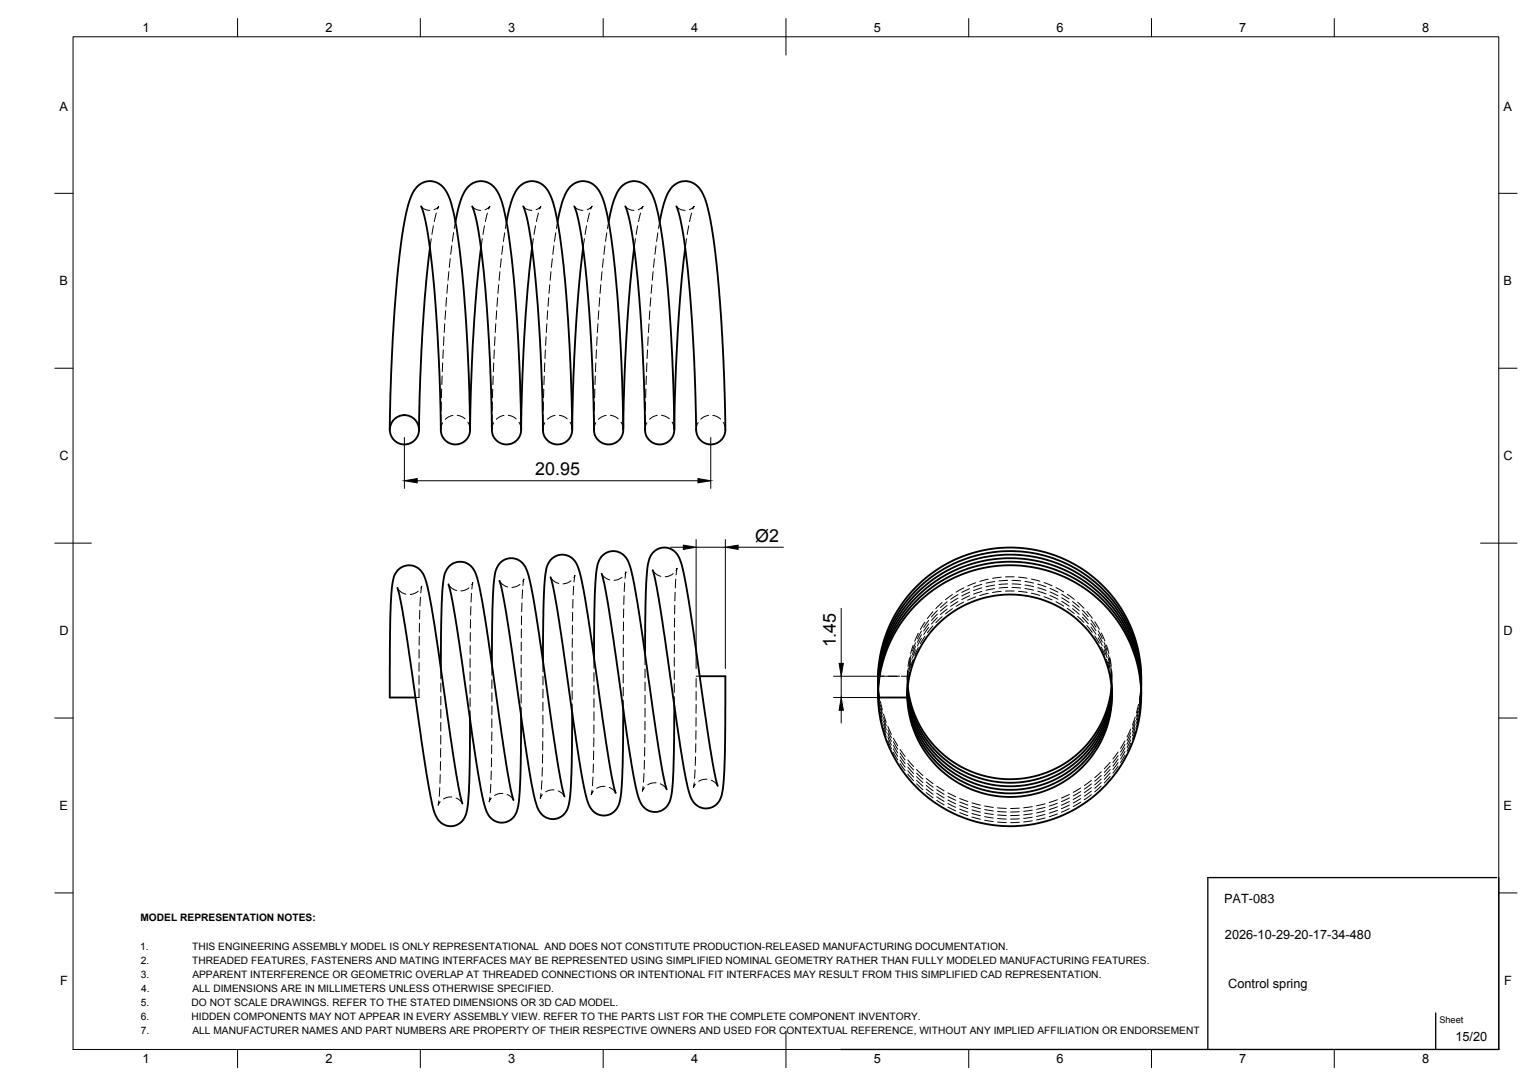
ISO-10303-21;
HEADER;
/* Generated by software containing ST-Developer
 * from STEP Tools, Inc. (www.steptools.com) 
 */

FILE_DESCRIPTION(
/* description */ ('PAT-083'),
/* implementation_level */ '2;1');

FILE_NAME(
/* name */ 'Control spring.step',
/* time_stamp */ '2026-10-29T20:18:00-07:00',
/* author */ (''),
/* organization */ (''),
/* preprocessor_version */ 'ST-DEVELOPER v20.2',
/* originating_system */ 'Autodesk Translation Framework v15.17.0.0',
/* authorisation */ '');

FILE_SCHEMA (('AUTOMOTIVE_DESIGN { 1 0 10303 214 3 1 1 }'));
ENDSEC;

DATA;
#10=MECHANICAL_DESIGN_GEOMETRIC_PRESENTATION_REPRESENTATION('',(#241),#8428);
#166=B_SPLINE_SURFACE_WITH_KNOTS('',3,3,((#7043,#7044,#7045,#7046,#7047,
#7048,#7049,#7050,#7051,#7052,#7053,#7054,#7055,#7056,#7057,#7058,#7059,
#7060,#7061,#7062,#7063,#7064,#7065,#7066,#7067,#7068,#7069,#7070,#7071,
#7072,#7073,#7074,#7075,#7076,#7077,#7078,#7079,#7080,#7081,#7082,#7083,
#7084,#7085,#7086,#7087,#7088,#7089,#7090,#7091,#7092,#7093,#7094,#7095,
#7096,#7097,#7098,#7099,#7100,#7101,#7102,#7103,#7104,#7105,#7106,#7107,
#7108,#7109,#7110,#7111,#7112,#7113),(#7114,#7115,#7116,#7117,#7118,#7119,
#7120,#7121,#7122,#7123,#7124,#7125,#7126,#7127,#7128,#7129,#7130,#7131,
#7132,#7133,#7134,#7135,#7136,#7137,#7138,#7139,#7140,#7141,#7142,#7143,
#7144,#7145,#7146,#7147,#7148,#7149,#7150,#7151,#7152,#7153,#7154,#7155,
#7156,#7157,#7158,#7159,#7160,#7161,#7162,#7163,#7164,#7165,#7166,#7167,
#7168,#7169,#7170,#7171,#7172,#7173,#7174,#7175,#7176,#7177,#7178,#7179,
#7180,#7181,#7182,#7183,#7184),(#7185,#7186,#7187,#7188,#7189,#7190,#7191,
#7192,#7193,#7194,#7195,#7196,#7197,#7198,#7199,#7200,#7201,#7202,#7203,
#7204,#7205,#7206,#7207,#7208,#7209,#7210,#7211,#7212,#7213,#7214,#7215,
#7216,#7217,#7218,#7219,#7220,#7221,#7222,#7223,#7224,#7225,#7226,#7227,
#7228,#7229,#7230,#7231,#7232,#7233,#7234,#7235,#7236,#7237,#7238,#7239,
#7240,#7241,#7242,#7243,#7244,#7245,#7246,#7247,#7248,#7249,#7250,#7251,
#7252,#7253,#7254,#7255),(#7256,#7257,#7258,#7259,#7260,#7261,#7262,#7263,
#7264,#7265,#7266,#7267,#7268,#7269,#7270,#7271,#7272,#7273,#7274,#7275,
#7276,#7277,#7278,#7279,#7280,#7281,#7282,#7283,#7284,#7285,#7286,#7287,
#7288,#7289,#7290,#7291,#7292,#7293,#7294,#7295,#7296,#7297,#7298,#7299,
#7300,#7301,#7302,#7303,#7304,#7305,#7306,#7307,#7308,#7309,#7310,#7311,
#7312,#7313,#7314,#7315,#7316,#7317,#7318,#7319,#7320,#7321,#7322,#7323,
#7324,#7325,#7326),(#7327,#7328,#7329,#7330,#7331,#7332,#7333,#7334,#7335,
#7336,#7337,#7338,#7339,#7340,#7341,#7342,#7343,#7344,#7345,#7346,#7347,
#7348,#7349,#7350,#7351,#7352,#7353,#7354,#7355,#7356,#7357,#7358,#7359,
#7360,#7361,#7362,#7363,#7364,#7365,#7366,#7367,#7368,#7369,#7370,#7371,
#7372,#7373,#7374,#7375,#7376,#7377,#7378,#7379,#7380,#7381,#7382,#7383,
#7384,#7385,#7386,#7387,#7388,#7389,#7390,#7391,#7392,#7393,#7394,#7395,
#7396,#7397),(#7398,#7399,#7400,#7401,#7402,#7403,#7404,#7405,#7406,#7407,
#7408,#7409,#7410,#7411,#7412,#7413,#7414,#7415,#7416,#7417,#7418,#7419,
#7420,#7421,#7422,#7423,#7424,#7425,#7426,#7427,#7428,#7429,#7430,#7431,
#7432,#7433,#7434,#7435,#7436,#7437,#7438,#7439,#7440,#7441,#7442,#7443,
#7444,#7445,#7446,#7447,#7448,#7449,#7450,#7451,#7452,#7453,#7454,#7455,
#7456,#7457,#7458,#7459,#7460,#7461,#7462,#7463,#7464,#7465,#7466,#7467,
#7468),(#7469,#7470,#7471,#7472,#7473,#7474,#7475,#7476,#7477,#7478,#7479,
#7480,#7481,#7482,#7483,#7484,#7485,#7486,#7487,#7488,#7489,#7490,#7491,
#7492,#7493,#7494,#7495,#7496,#7497,#7498,#7499,#7500,#7501,#7502,#7503,
#7504,#7505,#7506,#7507,#7508,#7509,#7510,#7511,#7512,#7513,#7514,#7515,
#7516,#7517,#7518,#7519,#7520,#7521,#7522,#7523,#7524,#7525,#7526,#7527,
#7528,#7529,#7530,#7531,#7532,#7533,#7534,#7535,#7536,#7537,#7538,#7539),
(#7540,#7541,#7542,#7543,#7544,#7545,#7546,#7547,#7548,#7549,#7550,#7551,
#7552,#7553,#7554,#7555,#7556,#7557,#7558,#7559,#7560,#7561,#7562,#7563,
#7564,#7565,#7566,#7567,#7568,#7569,#7570,#7571,#7572,#7573,#7574,#7575,
#7576,#7577,#7578,#7579,#7580,#7581,#7582,#7583,#7584,#7585,#7586,#7587,
#7588,#7589,#7590,#7591,#7592,#7593,#7594,#7595,#7596,#7597,#7598,#7599,
#7600,#7601,#7602,#7603,#7604,#7605,#7606,#7607,#7608,#7609,#7610),(#7611,
#7612,#7613,#7614,#7615,#7616,#7617,#7618,#7619,#7620,#7621,#7622,#7623,
#7624,#7625,#7626,#7627,#7628,#7629,#7630,#7631,#7632,#7633,#7634,#7635,
#7636,#7637,#7638,#7639,#7640,#7641,#7642,#7643,#7644,#7645,#7646,#7647,
#7648,#7649,#7650,#7651,#7652,#7653,#7654,#7655,#7656,#7657,#7658,#7659,
#7660,#7661,#7662,#7663,#7664,#7665,#7666,#7667,#7668,#7669,#7670,#7671,
#7672,#7673,#7674,#7675,#7676,#7677,#7678,#7679,#7680,#7681),(#7682,#7683,
#7684,#7685,#7686,#7687,#7688,#7689,#7690,#7691,#7692,#7693,#7694,#7695,
#7696,#7697,#7698,#7699,#7700,#7701,#7702,#7703,#7704,#7705,#7706,#7707,
#7708,#7709,#7710,#7711,#7712,#7713,#7714,#7715,#7716,#7717,#7718,#7719,
#7720,#7721,#7722,#7723,#7724,#7725,#7726,#7727,#7728,#7729,#7730,#7731,
#7732,#7733,#7734,#7735,#7736,#7737,#7738,#7739,#7740,#7741,#7742,#7743,
#7744,#7745,#7746,#7747,#7748,#7749,#7750,#7751,#7752)),.UNSPECIFIED.,.T.,
 .F.,.F.,(4,1,1,1,1,1,1,4),(4,1,1,1,1,1,1,1,1,1,1,1,1,1,1,1,1,1,1,1,1,1,
1,1,1,1,1,1,1,1,1,1,1,1,1,1,1,1,1,1,1,1,1,1,1,1,1,1,1,1,1,1,1,1,1,1,1,1,
1,1,1,1,1,1,1,1,1,1,4),(-3.14159265358979,-2.24399475256414,-1.34639685153848,
-0.448798950512828,0.448798950512828,1.34639685153848,2.24399475256414,
3.14159265358979),(0.,0.0178571428571429,0.0357142857142857,0.0535714285714286,
0.0714285714285714,0.0892857142857143,0.107142857142857,0.125,0.142857142857143,
0.150793650793651,0.158730158730159,0.174603174603175,0.19047619047619,
0.202380952380952,0.214285714285714,0.226190476190476,0.238095238095238,
0.25,0.261904761904762,0.267857142857143,0.273809523809524,0.285714285714286,
0.297619047619048,0.30952380952381,0.321428571428571,0.333333333333333,
0.349206349206349,0.365079365079365,0.380952380952381,0.396825396825397,
0.412698412698413,0.428571428571429,0.446428571428571,0.464285714285714,
0.476190476190476,0.488095238095238,0.5,0.517857142857143,0.535714285714286,
0.553571428571429,0.571428571428571,0.589285714285714,0.607142857142857,
0.625,0.642857142857143,0.660714285714286,0.678571428571428,0.696428571428571,
0.714285714285714,0.726190476190476,0.738095238095238,0.75,0.761904761904762,
0.773809523809524,0.785714285714286,0.797619047619047,0.809523809523809,
0.821428571428571,0.833333333333333,0.845238095238095,0.857142857142857,
0.875,0.892857142857143,0.910714285714286,0.928571428571429,0.946428571428571,
0.964285714285714,0.982142857142857,1.),.UNSPECIFIED.);
#177=B_SPLINE_CURVE_WITH_KNOTS('',3,(#7756,#7757,#7758,#7759,#7760,#7761,
#7762,#7763,#7764,#7765,#7766,#7767,#7768,#7769,#7770,#7771,#7772,#7773,
#7774,#7775,#7776,#7777,#7778,#7779,#7780,#7781,#7782,#7783,#7784,#7785,
#7786,#7787,#7788,#7789,#7790,#7791,#7792,#7793,#7794,#7795,#7796,#7797,
#7798,#7799,#7800,#7801,#7802,#7803,#7804,#7805,#7806,#7807,#7808,#7809,
#7810,#7811,#7812,#7813,#7814,#7815,#7816,#7817,#7818,#7819,#7820,#7821,
#7822,#7823,#7824,#7825,#7826),.UNSPECIFIED.,.F.,.F.,(4,1,1,1,1,1,1,1,1,
1,1,1,1,1,1,1,1,1,1,1,1,1,1,1,1,1,1,1,1,1,1,1,1,1,1,1,1,1,1,1,1,1,1,1,1,
1,1,1,1,1,1,1,1,1,1,1,1,1,1,1,1,1,1,1,1,1,1,1,4),(0.,0.0178571428571429,
0.0357142857142857,0.0535714285714286,0.0714285714285714,0.0892857142857143,
0.107142857142857,0.125,0.142857142857143,0.150793650793651,0.158730158730159,
0.174603174603175,0.19047619047619,0.202380952380952,0.214285714285714,
0.226190476190476,0.238095238095238,0.25,0.261904761904762,0.267857142857143,
0.273809523809524,0.285714285714286,0.297619047619048,0.30952380952381,
0.321428571428571,0.333333333333333,0.349206349206349,0.365079365079365,
0.380952380952381,0.396825396825397,0.412698412698413,0.428571428571429,
0.446428571428571,0.464285714285714,0.476190476190476,0.488095238095238,
0.5,0.517857142857143,0.535714285714286,0.553571428571429,0.571428571428571,
0.589285714285714,0.607142857142857,0.625,0.642857142857143,0.660714285714286,
0.678571428571428,0.696428571428571,0.714285714285714,0.726190476190476,
0.738095238095238,0.75,0.761904761904762,0.773809523809524,0.785714285714286,
0.797619047619047,0.809523809523809,0.821428571428571,0.833333333333333,
0.845238095238095,0.857142857142857,0.875,0.892857142857143,0.910714285714286,
0.928571428571429,0.946428571428571,0.964285714285714,0.982142857142857,
1.),.UNSPECIFIED.);
#193=SHAPE_REPRESENTATION_RELATIONSHIP('SRR','None',#8527,#217);
#217=ADVANCED_BREP_SHAPE_REPRESENTATION('',(#265),#8416);
#241=STYLED_ITEM('',(#8705),#265);
#265=MANIFOLD_SOLID_BREP('Body1',#3687);
#421=PLANE('',#4240);
#422=PLANE('',#4241);
#622=FACE_OUTER_BOUND('',#920,.T.);
#623=FACE_OUTER_BOUND('',#921,.T.);
#624=FACE_OUTER_BOUND('',#922,.T.);
#920=EDGE_LOOP('',(#2960,#2961,#2962,#2963));
#921=EDGE_LOOP('',(#2964));
#922=EDGE_LOOP('',(#2965));
#1662=CIRCLE('',#4238,0.1);
#1663=CIRCLE('',#4239,0.1);
#1875=VERTEX_POINT('',#7753);
#1876=VERTEX_POINT('',#7755);
#2256=EDGE_CURVE('',#1875,#1875,#1662,.T.);
#2257=EDGE_CURVE('',#1875,#1876,#177,.T.);
#2258=EDGE_CURVE('',#1876,#1876,#1663,.T.);
#2960=ORIENTED_EDGE('',*,*,#2256,.T.);
#2961=ORIENTED_EDGE('',*,*,#2257,.T.);
#2962=ORIENTED_EDGE('',*,*,#2258,.F.);
#2963=ORIENTED_EDGE('',*,*,#2257,.F.);
#2964=ORIENTED_EDGE('',*,*,#2258,.T.);
#2965=ORIENTED_EDGE('',*,*,#2256,.F.);
#3569=ADVANCED_FACE('',(#622),#166,.T.);
#3570=ADVANCED_FACE('',(#623),#421,.T.);
#3571=ADVANCED_FACE('',(#624),#422,.F.);
#3687=CLOSED_SHELL('',(#3569,#3570,#3571));
#4237=AXIS2_PLACEMENT_3D('',#7042,#5087,#5088);
#4238=AXIS2_PLACEMENT_3D('',#7754,#5089,#5090);
#4239=AXIS2_PLACEMENT_3D('',#7827,#5091,#5092);
#4240=AXIS2_PLACEMENT_3D('',#7828,#5093,#5094);
#4241=AXIS2_PLACEMENT_3D('',#7829,#5095,#5096);
#5087=DIRECTION('axis',(0.,0.,1.));
#5088=DIRECTION('refdir',(1.,0.,0.));
#5089=DIRECTION('center_axis',(-0.000134591856444243,0.997598919682403,
0.0692558830247305));
#5090=DIRECTION('ref_axis',(9.34371278597603E-6,-0.0692558823944232,0.997598928761687));
#5091=DIRECTION('center_axis',(0.000134591670588553,0.997598919668532,0.0692558832248945));
#5092=DIRECTION('ref_axis',(-0.499431472094232,0.0600671278230296,-0.864268560597272));
#5093=DIRECTION('center_axis',(0.000134591670588553,0.997598919668532,0.0692558832248945));
#5094=DIRECTION('ref_axis',(-0.499431472094232,0.0600671278230296,-0.864268560597272));
#5095=DIRECTION('center_axis',(-0.000134591856444243,0.997598919682403,
0.0692558830247305));
#5096=DIRECTION('ref_axis',(9.34371278597603E-6,-0.0692558823944232,0.997598928761687));
#7042=CARTESIAN_POINT('',(0.,0.,0.));
#7043=CARTESIAN_POINT('Ctrl Pts',(0.799999065628721,0.00692558823944229,
5.30024010712383));
#7044=CARTESIAN_POINT('Ctrl Pts',(0.799974755250737,0.187114846749742,5.31274930893178));
#7045=CARTESIAN_POINT('Ctrl Pts',(0.674578200671659,0.546127076651831,5.33781512365923));
#7046=CARTESIAN_POINT('Ctrl Pts',(0.187998995393781,0.852903359039399,5.37564381521248));
#7047=CARTESIAN_POINT('Ctrl Pts',(-0.386721866921525,0.788448388841122,
5.41368605209984));
#7048=CARTESIAN_POINT('Ctrl Pts',(-0.7983994419892,0.377627224111744,5.45194644400096));
#7049=CARTESIAN_POINT('Ctrl Pts',(-0.864375113399524,-0.203617876612744,
5.49042055747836));
#7050=CARTESIAN_POINT('Ctrl Pts',(-0.552019639313923,-0.701812288635587,
5.52910737914477));
#7051=CARTESIAN_POINT('Ctrl Pts',(0.00615426428515267,-0.897757418326962,
5.56800374230524));
#7052=CARTESIAN_POINT('Ctrl Pts',(0.463089276607972,-0.737891299975203,
5.59986549204054));
#7053=CARTESIAN_POINT('Ctrl Pts',(0.706662565433678,-0.474149107376678,
5.62457829573124));
#7054=CARTESIAN_POINT('Ctrl Pts',(0.854347338563578,-0.169471123140589,
5.6478904398873));
#7055=CARTESIAN_POINT('Ctrl Pts',(0.854381411403854,0.269671075667267,5.67712918390586));
#7056=CARTESIAN_POINT('Ctrl Pts',(0.581578462406747,0.670744438556907,5.70943359497258));
#7057=CARTESIAN_POINT('Ctrl Pts',(0.189982000930166,0.858805851522918,5.73891161848027));
#7058=CARTESIAN_POINT('Ctrl Pts',(-0.201854620920769,0.859148371452269,
5.76552549972421));
#7059=CARTESIAN_POINT('Ctrl Pts',(-0.556170302204947,0.688486751453872,
5.79222147180784));
#7060=CARTESIAN_POINT('Ctrl Pts',(-0.802120584542054,0.380288702719923,
5.81899788702529));
#7061=CARTESIAN_POINT('Ctrl Pts',(-0.890321102734134,-0.0053444036833259,
5.84585301727138));
#7062=CARTESIAN_POINT('Ctrl Pts',(-0.816781798992104,-0.327577127496462,
5.86829638740099));
#7063=CARTESIAN_POINT('Ctrl Pts',(-0.678277859648778,-0.547664335405585,
5.88628859994389));
#7064=CARTESIAN_POINT('Ctrl Pts',(-0.494316135451619,-0.731945478665225,
5.90430550175064));
#7065=CARTESIAN_POINT('Ctrl Pts',(-0.194941007989142,-0.876310026230692,
5.92687230420244));
#7066=CARTESIAN_POINT('Ctrl Pts',(0.204945568353256,-0.876409485122255,
5.95402353339188));
#7067=CARTESIAN_POINT('Ctrl Pts',(0.566325487118899,-0.702556101088839,
5.98124373289334));
#7068=CARTESIAN_POINT('Ctrl Pts',(0.816751045229916,-0.388463305588866,
6.00853075028047));
#7069=CARTESIAN_POINT('Ctrl Pts',(0.917174982875959,0.0480250206861584,
6.03892142694837));
#7070=CARTESIAN_POINT('Ctrl Pts',(0.768829350780382,0.528866010776267,6.07244001895545));
#7071=CARTESIAN_POINT('Ctrl Pts',(0.338627495917749,0.872873034891815,6.10911095186911));
#7072=CARTESIAN_POINT('Ctrl Pts',(-0.212178222814091,0.914151313349766,
6.14588130840082));
#7073=CARTESIAN_POINT('Ctrl Pts',(-0.691759933067223,0.637451614256161,
6.18274515756461));
#7074=CARTESIAN_POINT('Ctrl Pts',(-0.932934482256533,0.137697594997002,
6.21969639210087));
#7075=CARTESIAN_POINT('Ctrl Pts',(-0.84730393945114,-0.435496308403701,
6.25827178793966));
#7076=CARTESIAN_POINT('Ctrl Pts',(-0.415273257958933,-0.868240176171726,
6.29847623644814));
#7077=CARTESIAN_POINT('Ctrl Pts',(0.146189896678077,-0.930950222024402,
6.33566388079779));
#7078=CARTESIAN_POINT('Ctrl Pts',(0.578787425776111,-0.722091726547751,
6.36825221458814));
#7079=CARTESIAN_POINT('Ctrl Pts',(0.835229259505866,-0.400278931762148,
6.3962159259868));
#7080=CARTESIAN_POINT('Ctrl Pts',(0.943177486850013,0.0688606453452641,
6.42887288667825));
#7081=CARTESIAN_POINT('Ctrl Pts',(0.756462512495389,0.604750444420971,6.46623690685835));
#7082=CARTESIAN_POINT('Ctrl Pts',(0.214509054547464,0.945343920852135,6.50831791566041));
#7083=CARTESIAN_POINT('Ctrl Pts',(-0.421585054233784,0.873670673138226,
6.55043539297339));
#7084=CARTESIAN_POINT('Ctrl Pts',(-0.874725713994987,0.420703846750279,
6.59257924943873));
#7085=CARTESIAN_POINT('Ctrl Pts',(-0.946491736933492,-0.216206220818672,
6.63473932973225));
#7086=CARTESIAN_POINT('Ctrl Pts',(-0.605472064685913,-0.758979181442101,
6.67690544450194));
#7087=CARTESIAN_POINT('Ctrl Pts',(-0.000509641250504898,-0.970641038681315,
6.71906739492544));
#7088=CARTESIAN_POINT('Ctrl Pts',(0.604236817182525,-0.758999928674301,
6.76121498571335));
#7089=CARTESIAN_POINT('Ctrl Pts',(0.944676427167983,-0.216670516455945,
6.80333805746961));
#7090=CARTESIAN_POINT('Ctrl Pts',(0.873719648783539,0.418956634979468,6.8454265042638));
#7091=CARTESIAN_POINT('Ctrl Pts',(0.421037273012308,0.871132652579719,6.88747029453994));
#7092=CARTESIAN_POINT('Ctrl Pts',(-0.142342851291253,0.933831870869633,
6.92479402146672));
#7093=CARTESIAN_POINT('Ctrl Pts',(-0.575104466317865,0.724476767443434,
6.95741054274359));
#7094=CARTESIAN_POINT('Ctrl Pts',(-0.831597121038275,0.403171008458228,
6.98533606563364));
#7095=CARTESIAN_POINT('Ctrl Pts',(-0.922808904665035,0.00254068286457492,
7.01322724854536));
#7096=CARTESIAN_POINT('Ctrl Pts',(-0.831484359832733,-0.397369041930912,
7.04108128388358));
#7097=CARTESIAN_POINT('Ctrl Pts',(-0.576024516479058,-0.717622866946566,
7.06889539860548));
#7098=CARTESIAN_POINT('Ctrl Pts',(-0.207464718971416,-0.895095126308869,
7.09666685370961));
#7099=CARTESIAN_POINT('Ctrl Pts',(0.200869050822812,-0.894893573965507,
7.12439296344474));
#7100=CARTESIAN_POINT('Ctrl Pts',(0.568135301656786,-0.717941543510051,
7.15207107099507));
#7101=CARTESIAN_POINT('Ctrl Pts',(0.821742493579341,-0.399813712939291,
7.17969857736332));
#7102=CARTESIAN_POINT('Ctrl Pts',(0.912100647381109,-0.00372699171446918,
7.20727292857109));
#7103=CARTESIAN_POINT('Ctrl Pts',(0.821667160899362,0.391120281113409,7.23479162069698));
#7104=CARTESIAN_POINT('Ctrl Pts',(0.527798142032111,0.760706416566583,7.26682897888736));
#7105=CARTESIAN_POINT('Ctrl Pts',(0.00437094025093319,0.944184514671381,
7.30334225024583));
#7106=CARTESIAN_POINT('Ctrl Pts',(-0.583164611559206,0.738086874931468,
7.3442757526392));
#7107=CARTESIAN_POINT('Ctrl Pts',(-0.912546668924433,0.213026529714121,
7.38505770065783));
#7108=CARTESIAN_POINT('Ctrl Pts',(-0.843060529623956,-0.400706652853849,
7.42568118182012));
#7109=CARTESIAN_POINT('Ctrl Pts',(-0.407835437985135,-0.835237258109269,
7.46613873367218));
#7110=CARTESIAN_POINT('Ctrl Pts',(0.200737244244076,-0.903598468057941,
7.5064251969444));
#7111=CARTESIAN_POINT('Ctrl Pts',(0.71672352100227,-0.578479045751934,7.54653146106904));
#7112=CARTESIAN_POINT('Ctrl Pts',(0.849917343436364,-0.197265324952655,
7.57314919120958));
#7113=CARTESIAN_POINT('Ctrl Pts',(0.849943147209423,-0.00600671278230411,
7.58642685605973));
#7114=CARTESIAN_POINT('Ctrl Pts',(0.770079135866838,0.00692155156817904,
5.30024010712383));
#7115=CARTESIAN_POINT('Ctrl Pts',(0.770055720112496,0.180479832525886,5.31228896941391));
#7116=CARTESIAN_POINT('Ctrl Pts',(0.649347137055222,0.526118956744516,5.33641790275693));
#7117=CARTESIAN_POINT('Ctrl Pts',(0.180677599950648,0.821679099419469,5.37285586761231));
#7118=CARTESIAN_POINT('Ctrl Pts',(-0.373128354027995,0.759596327571503,
5.40950951731212));
#7119=CARTESIAN_POINT('Ctrl Pts',(-0.770051450984494,0.363580245990391,
5.44639246645647));
#7120=CARTESIAN_POINT('Ctrl Pts',(-0.833750732775199,-0.197081341774288,
5.48350071817735));
#7121=CARTESIAN_POINT('Ctrl Pts',(-0.532331315046715,-0.677969641751496,
5.5208364575171));
#7122=CARTESIAN_POINT('Ctrl Pts',(0.00675318837749655,-0.867294541965757,
5.558400781988));
#7123=CARTESIAN_POINT('Ctrl Pts',(0.448424688054875,-0.712845112569316,
5.58919119813692));
#7124=CARTESIAN_POINT('Ctrl Pts',(0.684012778929899,-0.457765801730765,
5.61309167265538));
#7125=CARTESIAN_POINT('Ctrl Pts',(0.82691455168644,-0.162993811747473,5.6356443242608));
#7126=CARTESIAN_POINT('Ctrl Pts',(0.82699649983482,0.262124971545771,5.66394696022895));
#7127=CARTESIAN_POINT('Ctrl Pts',(0.562750276158912,0.650752034831193,5.69524212629919));
#7128=CARTESIAN_POINT('Ctrl Pts',(0.183080725565527,0.833119661747386,5.72381920452852));
#7129=CARTESIAN_POINT('Ctrl Pts',(-0.197084703463694,0.833490239824234,
5.74963623066415));
#7130=CARTESIAN_POINT('Ctrl Pts',(-0.541119975074503,0.667809968168665,
5.77555492059187));
#7131=CARTESIAN_POINT('Ctrl Pts',(-0.780113947482257,0.368392103745768,
5.80156649252668));
#7132=CARTESIAN_POINT('Ctrl Pts',(-0.865905134963049,-0.00656170868815412,
5.82767483842523));
#7133=CARTESIAN_POINT('Ctrl Pts',(-0.794375852743549,-0.320111204417347,
5.84950881094256));
#7134=CARTESIAN_POINT('Ctrl Pts',(-0.659521269028743,-0.534410811061921,
5.86702622272765));
#7135=CARTESIAN_POINT('Ctrl Pts',(-0.480335340635082,-0.713917263728105,
5.88457460840773));
#7136=CARTESIAN_POINT('Ctrl Pts',(-0.188587087034294,-0.854642083096481,
5.90656315000717));
#7137=CARTESIAN_POINT('Ctrl Pts',(0.201462529249485,-0.854779640403169,
5.9330427097564));
#7138=CARTESIAN_POINT('Ctrl Pts',(0.554262072476138,-0.685098200004362,
5.95961046024728));
#7139=CARTESIAN_POINT('Ctrl Pts',(0.798967352085236,-0.378235706832728,
5.98626742358202));
#7140=CARTESIAN_POINT('Ctrl Pts',(0.89721847916451,0.0485845903033819,6.01597993297972));
#7141=CARTESIAN_POINT('Ctrl Pts',(0.752070839701578,0.519313731169816,6.04878757680353));
#7142=CARTESIAN_POINT('Ctrl Pts',(0.330497979661169,0.856564661134425,6.08472490306161));
#7143=CARTESIAN_POINT('Ctrl Pts',(-0.209973066601811,0.897165035883339,
6.12079612560753));
#7144=CARTESIAN_POINT('Ctrl Pts',(-0.68120970786282,0.625397209779933,6.15700765884533));
#7145=CARTESIAN_POINT('Ctrl Pts',(-0.918572438612158,0.13378828614086,6.19335554838198));
#7146=CARTESIAN_POINT('Ctrl Pts',(-0.83433799028855,-0.430850802296383,
6.23134861625561));
#7147=CARTESIAN_POINT('Ctrl Pts',(-0.408316865658928,-0.857793214073537,
6.2709938323838));
#7148=CARTESIAN_POINT('Ctrl Pts',(0.146288162282126,-0.919868958459814,
6.30771962173879));
#7149=CARTESIAN_POINT('Ctrl Pts',(0.574223288772557,-0.71333190916663,6.33995134748923));
#7150=CARTESIAN_POINT('Ctrl Pts',(0.828161465810104,-0.394717048019018,
6.36763553346922));
#7151=CARTESIAN_POINT('Ctrl Pts',(0.935214831817973,0.0702367246280078,
6.39999872706231));
#7152=CARTESIAN_POINT('Ctrl Pts',(0.750063250540666,0.602049612066996,6.43706602732403));
#7153=CARTESIAN_POINT('Ctrl Pts',(0.211520380136952,0.940697836629915,6.47888152979277));
#7154=CARTESIAN_POINT('Ctrl Pts',(-0.421676436247289,0.869510362169926,
6.52079671898647));
#7155=CARTESIAN_POINT('Ctrl Pts',(-0.873553921061096,0.418039168812721,
6.56280406058959));
#7156=CARTESIAN_POINT('Ctrl Pts',(-0.945379508760524,-0.217899113421901,
6.60489250808515));
#7157=CARTESIAN_POINT('Ctrl Pts',(-0.604485708962148,-0.760787236561161,
6.64705240063428));
#7158=CARTESIAN_POINT('Ctrl Pts',(0.00138176225817566,-0.972945250150102,
6.6892731978663));
#7159=CARTESIAN_POINT('Ctrl Pts',(0.608080140735397,-0.760798630125154,
6.73154461863783));
#7160=CARTESIAN_POINT('Ctrl Pts',(0.950239792824421,-0.216025881173973,
6.77385551750453));
#7161=CARTESIAN_POINT('Ctrl Pts',(0.879017289772042,0.423590907490335,6.81620268596198));
#7162=CARTESIAN_POINT('Ctrl Pts',(0.422960901581898,0.879362908068112,6.85856017311708));
#7163=CARTESIAN_POINT('Ctrl Pts',(-0.145593093231334,0.942790559668914,
6.89621968364161));
#7164=CARTESIAN_POINT('Ctrl Pts',(-0.582932490358213,0.73127758858104,6.92917512678282));
#7165=CARTESIAN_POINT('Ctrl Pts',(-0.842401988544835,0.406320842666593,
6.957415448388));
#7166=CARTESIAN_POINT('Ctrl Pts',(-0.934795701286156,0.000685604828614038,
6.985653769321));
#7167=CARTESIAN_POINT('Ctrl Pts',(-0.842294766840471,-0.404603381671274,
7.01387715318084));
#7168=CARTESIAN_POINT('Ctrl Pts',(-0.583187447906784,-0.729494778082508,
7.04208836805485));
#7169=CARTESIAN_POINT('Ctrl Pts',(-0.20899792340701,-0.909726737101999,
7.07028057033796));
#7170=CARTESIAN_POINT('Ctrl Pts',(0.206012719667752,-0.909558569724805,
7.09845804612497));
#7171=CARTESIAN_POINT('Ctrl Pts',(0.579624839727756,-0.72959465407811,7.12660922044297));
#7172=CARTESIAN_POINT('Ctrl Pts',(0.837867106227739,-0.405711083857505,
7.15473493621397));
#7173=CARTESIAN_POINT('Ctrl Pts',(0.929983985732294,-0.00207542308664412,
7.18283200361311));
#7174=CARTESIAN_POINT('Ctrl Pts',(0.837775922394786,0.40066931879227,7.21089711007051));
#7175=CARTESIAN_POINT('Ctrl Pts',(0.537807840870324,0.777996358577212,7.24360025784798));
#7176=CARTESIAN_POINT('Ctrl Pts',(0.00294143852372089,0.965597941956312,
7.28090792189502));
#7177=CARTESIAN_POINT('Ctrl Pts',(-0.59827790503141,0.754837569025208,7.32278668150169));
#7178=CARTESIAN_POINT('Ctrl Pts',(-0.935814946990508,0.217001877726337,
7.36456027598379));
#7179=CARTESIAN_POINT('Ctrl Pts',(-0.864667175323564,-0.412475523451113,
7.40622093849563));
#7180=CARTESIAN_POINT('Ctrl Pts',(-0.417866766747618,-0.858729006758795,
7.44775776125507));
#7181=CARTESIAN_POINT('Ctrl Pts',(0.207655975088153,-0.929085997388315,
7.48916462895728));
#7182=CARTESIAN_POINT('Ctrl Pts',(0.73862266392267,-0.594662305466805,7.53042707168622));
#7183=CARTESIAN_POINT('Ctrl Pts',(0.875837799539084,-0.201989676969171,
7.55784229424685));
#7184=CARTESIAN_POINT('Ctrl Pts',(0.875864379853922,-0.00497530564290791,
7.5715195387037));
#7185=CARTESIAN_POINT('Ctrl Pts',(0.710428941733949,0.00492953088558486,
5.32881831830437));
#7186=CARTESIAN_POINT('Ctrl Pts',(0.71040731614315,0.165219065394011,5.33994603008611));
#7187=CARTESIAN_POINT('Ctrl Pts',(0.599024128589712,0.483870366740507,5.3621924509196));
#7188=CARTESIAN_POINT('Ctrl Pts',(0.167205166996449,0.75612127364975,5.39576440291455));
#7189=CARTESIAN_POINT('Ctrl Pts',(-0.342469011252512,0.698867316238289,
5.42949607339388));
#7190=CARTESIAN_POINT('Ctrl Pts',(-0.707447256311363,0.334638873927445,
5.46341601587375));
#7191=CARTESIAN_POINT('Ctrl Pts',(-0.765942731942805,-0.180685845273631,
5.49752276624412));
#7192=CARTESIAN_POINT('Ctrl Pts',(-0.488977975671522,-0.622493468082251,
5.53182729600019));
#7193=CARTESIAN_POINT('Ctrl Pts',(0.00623870066985125,-0.79639957834953,
5.56633555615365));
#7194=CARTESIAN_POINT('Ctrl Pts',(0.411979748797062,-0.65451285296037,5.59462344155862));
#7195=CARTESIAN_POINT('Ctrl Pts',(0.628431910779513,-0.420156210117234,
5.61658281146561));
#7196=CARTESIAN_POINT('Ctrl Pts',(0.759739764112401,-0.149292484888909,
5.63730747934422));
#7197=CARTESIAN_POINT('Ctrl Pts',(0.759837930575591,0.241447639232068,5.66332246132793));
#7198=CARTESIAN_POINT('Ctrl Pts',(0.516864570620339,0.598828714990839,5.6921027083035));
#7199=CARTESIAN_POINT('Ctrl Pts',(0.16754402090728,0.766642660816134,5.7183984452765));
#7200=CARTESIAN_POINT('Ctrl Pts',(-0.18243289406626,0.766996703299491,5.74216819224318));
#7201=CARTESIAN_POINT('Ctrl Pts',(-0.499344694617947,0.614409373974203,
5.7660436717059));
#7202=CARTESIAN_POINT('Ctrl Pts',(-0.719666388043044,0.338417073722969,
5.79002421526266));
#7203=CARTESIAN_POINT('Ctrl Pts',(-0.798838486989696,-0.00747184320142611,
5.81411179267834));
#7204=CARTESIAN_POINT('Ctrl Pts',(-0.732821087254027,-0.296979929993814,
5.83427424859502));
#7205=CARTESIAN_POINT('Ctrl Pts',(-0.608236501384017,-0.494969333219339,
5.85045910955365));
#7206=CARTESIAN_POINT('Ctrl Pts',(-0.442617486739659,-0.660891288693568,
5.8666802534398));
#7207=CARTESIAN_POINT('Ctrl Pts',(-0.172748327050428,-0.791093551297648,
5.88702427548063));
#7208=CARTESIAN_POINT('Ctrl Pts',(0.188434824933959,-0.791259517626132,
5.91154722254856));
#7209=CARTESIAN_POINT('Ctrl Pts',(0.515509148139609,-0.63399975107043,5.93618028019028));
#7210=CARTESIAN_POINT('Ctrl Pts',(0.742660619778638,-0.349226128508519,
5.96092404661359));
#7211=CARTESIAN_POINT('Ctrl Pts',(0.834013573979388,0.047387173011833,5.98854018010049));
#7212=CARTESIAN_POINT('Ctrl Pts',(0.699054298781812,0.485509196729349,6.01907630606175));
#7213=CARTESIAN_POINT('Ctrl Pts',(0.306089489608805,0.800037047528466,6.05258598067156));
#7214=CARTESIAN_POINT('Ctrl Pts',(-0.198806257075136,0.83811783046203,6.08629244673437));
#7215=CARTESIAN_POINT('Ctrl Pts',(-0.639994604888811,0.58386009688861,6.12019546148202));
#7216=CARTESIAN_POINT('Ctrl Pts',(-0.862778510831916,0.122809110352501,
6.15429381358228));
#7217=CARTESIAN_POINT('Ctrl Pts',(-0.783768475044449,-0.408002461396071,
6.19001514975991));
#7218=CARTESIAN_POINT('Ctrl Pts',(-0.382461984654271,-0.810530499122485,
6.22738726758261));
#7219=CARTESIAN_POINT('Ctrl Pts',(0.141571880318707,-0.869426431241229,
6.26209856247513));
#7220=CARTESIAN_POINT('Ctrl Pts',(0.546857792365987,-0.673923824775829,
6.29262411862805));
#7221=CARTESIAN_POINT('Ctrl Pts',(0.787850231799947,-0.371686474029746,
6.31889326617887));
#7222=CARTESIAN_POINT('Ctrl Pts',(0.889701212277186,0.0702541647771362,
6.34966096595927));
#7223=CARTESIAN_POINT('Ctrl Pts',(0.713512875154728,0.577124702757749,6.38499463961466));
#7224=CARTESIAN_POINT('Ctrl Pts',(0.198967909509621,0.901053551471294,6.42496855240101));
#7225=CARTESIAN_POINT('Ctrl Pts',(-0.408089575093021,0.833131022176632,
6.46516128973043));
#7226=CARTESIAN_POINT('Ctrl Pts',(-0.842862380754781,0.399211540997894,
6.50556671739343));
#7227=CARTESIAN_POINT('Ctrl Pts',(-0.912482057616401,-0.214227019813974,
6.54617863195434));
#7228=CARTESIAN_POINT('Ctrl Pts',(-0.582857572239619,-0.739804921207224,
6.58699019870486));
#7229=CARTESIAN_POINT('Ctrl Pts',(0.00529210032697009,-0.946120388887076,
6.62799422182894));
#7230=CARTESIAN_POINT('Ctrl Pts',(0.596417413889089,-0.73978975515068,6.66918308377763));
#7231=CARTESIAN_POINT('Ctrl Pts',(0.931157121946736,-0.20751322428765,6.71054882574604));
#7232=CARTESIAN_POINT('Ctrl Pts',(0.861650483779265,0.419727599707763,6.75208097200662));
#7233=CARTESIAN_POINT('Ctrl Pts',(0.413147604956643,0.868498049400113,6.79377525221771));
#7234=CARTESIAN_POINT('Ctrl Pts',(-0.148210983168275,0.931421962876526,
6.83097036528324));
#7235=CARTESIAN_POINT('Ctrl Pts',(-0.581294729795694,0.722118347875597,
6.86360544825447));
#7236=CARTESIAN_POINT('Ctrl Pts',(-0.838871906802363,0.399682199015836,
6.89163933377065));
#7237=CARTESIAN_POINT('Ctrl Pts',(-0.930877231252504,-0.00373870819751691,
6.91972773631357));
#7238=CARTESIAN_POINT('Ctrl Pts',(-0.838749751075799,-0.407817095097561,
6.94787183402895));
#7239=CARTESIAN_POINT('Ctrl Pts',(-0.579931993725618,-0.732521582072749,
6.9760659349542));
#7240=CARTESIAN_POINT('Ctrl Pts',(-0.205212822112969,-0.913124822787424,
7.00430873475179));
#7241=CARTESIAN_POINT('Ctrl Pts',(0.211338054228992,-0.913070414334495,
7.03259350527625));
#7242=CARTESIAN_POINT('Ctrl Pts',(0.587263134138024,-0.732110657981568,
7.06092123472863));
#7243=CARTESIAN_POINT('Ctrl Pts',(0.847742099102453,-0.405599817717801,
7.08928670598057));
#7244=CARTESIAN_POINT('Ctrl Pts',(0.940948978785284,0.00228770078596691,
7.1176867396323));
#7245=CARTESIAN_POINT('Ctrl Pts',(0.847659354457111,0.410238520315532,7.14611819660086));
#7246=CARTESIAN_POINT('Ctrl Pts',(0.543275903219406,0.793339172582683,7.17932027275837));
#7247=CARTESIAN_POINT('Ctrl Pts',(-0.001093578869141,0.984623315384901,
7.21730924712761));
#7248=CARTESIAN_POINT('Ctrl Pts',(-0.615252284949225,0.769726133995085,
7.26008973650359));
#7249=CARTESIAN_POINT('Ctrl Pts',(-0.961422256849412,0.218820343216691,
7.30290266259028));
#7250=CARTESIAN_POINT('Ctrl Pts',(-0.888633848724617,-0.428292780832149,
7.34573759998394));
#7251=CARTESIAN_POINT('Ctrl Pts',(-0.42811642962634,-0.888746898872104,
7.38857936211361));
#7252=CARTESIAN_POINT('Ctrl Pts',(0.218959376739582,-0.961833511797225,
7.43142516328682));
#7253=CARTESIAN_POINT('Ctrl Pts',(0.770122900311167,-0.615157339727794,
7.47424382285298));
#7254=CARTESIAN_POINT('Ctrl Pts',(0.913207865694905,-0.206388594750497,
7.5027957331042));
#7255=CARTESIAN_POINT('Ctrl Pts',(0.913235549072487,-0.00119827763899913,
7.51704057274925));
#7256=CARTESIAN_POINT('Ctrl Pts',(0.688502394196997,-0.00177585944161231,
5.42536374837757));
#7257=CARTESIAN_POINT('Ctrl Pts',(0.688481448875166,0.153471500858794,5.43614141945633));
#7258=CARTESIAN_POINT('Ctrl Pts',(0.580508040541705,0.46124670025465,5.45764245524231));
#7259=CARTESIAN_POINT('Ctrl Pts',(0.165662319023174,0.722161337503787,5.48987538957648));
#7260=CARTESIAN_POINT('Ctrl Pts',(-0.320578571387279,0.667050889553626,
5.52206618528612));
#7261=CARTESIAN_POINT('Ctrl Pts',(-0.666378826232044,0.32127882597957,5.55424091986707));
#7262=CARTESIAN_POINT('Ctrl Pts',(-0.721063694800031,-0.164642450695304,
5.58640440743116));
#7263=CARTESIAN_POINT('Ctrl Pts',(-0.461013415699651,-0.578597703078686,
5.61857188153771));
#7264=CARTESIAN_POINT('Ctrl Pts',(0.000868763121645957,-0.740322038056404,
5.65075229330461));
#7265=CARTESIAN_POINT('Ctrl Pts',(0.377087016267437,-0.608394442936668,
5.67699673395361));
#7266=CARTESIAN_POINT('Ctrl Pts',(0.577057627822796,-0.391810817241549,
5.69729012722977));
#7267=CARTESIAN_POINT('Ctrl Pts',(0.698092236754842,-0.142020837867168,
5.71640197572506));
#7268=CARTESIAN_POINT('Ctrl Pts',(0.697963439505406,0.21710900600399,5.74031529151263));
#7269=CARTESIAN_POINT('Ctrl Pts',(0.475355133020151,0.544099194249106,5.76666169992576));
#7270=CARTESIAN_POINT('Ctrl Pts',(0.156654851678278,0.697080460332168,5.79065302227195));
#7271=CARTESIAN_POINT('Ctrl Pts',(-0.161711917448867,0.697304453295988,
5.81227877536069));
#7272=CARTESIAN_POINT('Ctrl Pts',(-0.449161842092396,0.558802207686871,
5.83393922469739));
#7273=CARTESIAN_POINT('Ctrl Pts',(-0.648454473279016,0.309008113535057,
5.85564132087709));
#7274=CARTESIAN_POINT('Ctrl Pts',(-0.719837707005216,-0.00322310267600228,
5.8773860839056));
#7275=CARTESIAN_POINT('Ctrl Pts',(-0.660324209075774,-0.263926195140504,
5.89554604949557));
#7276=CARTESIAN_POINT('Ctrl Pts',(-0.548312630732919,-0.441913047209008,
5.91009721234879));
#7277=CARTESIAN_POINT('Ctrl Pts',(-0.399568209162923,-0.590912445741052,
5.92466534563453));
#7278=CARTESIAN_POINT('Ctrl Pts',(-0.157550820881924,-0.70761172499092,
5.94291010238594));
#7279=CARTESIAN_POINT('Ctrl Pts',(0.165683821816319,-0.707692893763189,
5.96485832442363));
#7280=CARTESIAN_POINT('Ctrl Pts',(0.457834734757014,-0.567156151977817,
5.98686542599537));
#7281=CARTESIAN_POINT('Ctrl Pts',(0.660365135739603,-0.313163685177989,
6.00893343132688));
#7282=CARTESIAN_POINT('Ctrl Pts',(0.741647053339758,0.0400023925443897,
6.03352542353788));
#7283=CARTESIAN_POINT('Ctrl Pts',(0.6215856897095,0.429424608756888,6.0606712019436));
#7284=CARTESIAN_POINT('Ctrl Pts',(0.272788863259715,0.708464025234,6.09040985442785));
#7285=CARTESIAN_POINT('Ctrl Pts',(-0.174640201386968,0.742128787355836,
6.12028246378202));
#7286=CARTESIAN_POINT('Ctrl Pts',(-0.565102038705666,0.517026489502915,
6.1502917775661));
#7287=CARTESIAN_POINT('Ctrl Pts',(-0.762043624567604,0.109327312662896,
6.18044350600909));
#7288=CARTESIAN_POINT('Ctrl Pts',(-0.692189456122551,-0.359678326088431,
6.21200701480215));
#7289=CARTESIAN_POINT('Ctrl Pts',(-0.337773460931687,-0.715129603852559,
6.24501197076816));
#7290=CARTESIAN_POINT('Ctrl Pts',(0.124866016940657,-0.767119798247897,
6.27565761479799));
#7291=CARTESIAN_POINT('Ctrl Pts',(0.482663833907203,-0.594530247737682,
6.30260654020584));
#7292=CARTESIAN_POINT('Ctrl Pts',(0.695450511759543,-0.32768100442103,6.32580056862507));
#7293=CARTESIAN_POINT('Ctrl Pts',(0.785412896461935,0.0626075158038052,
6.35297268106789));
#7294=CARTESIAN_POINT('Ctrl Pts',(0.629799785153589,0.510459438093438,6.38419099540486));
#7295=CARTESIAN_POINT('Ctrl Pts',(0.174872432500897,0.796962684150136,6.41953687685404));
#7296=CARTESIAN_POINT('Ctrl Pts',(-0.362484676752387,0.736952725256016,
6.4551134881321));
#7297=CARTESIAN_POINT('Ctrl Pts',(-0.74792746534711,0.35245915978463,6.49092474388711));
#7298=CARTESIAN_POINT('Ctrl Pts',(-0.809887309570728,-0.192065947901566,
6.52697449126839));
#7299=CARTESIAN_POINT('Ctrl Pts',(-0.516915158076634,-0.65954619222211,
6.56326583721123));
#7300=CARTESIAN_POINT('Ctrl Pts',(0.00709632936792426,-0.843579839117015,
6.59980147205316));
#7301=CARTESIAN_POINT('Ctrl Pts',(0.535080054211952,-0.659528972736876,
6.63658345012356));
#7302=CARTESIAN_POINT('Ctrl Pts',(0.834961098454938,-0.183143056575008,
6.67361341976074));
#7303=CARTESIAN_POINT('Ctrl Pts',(0.772836475154942,0.379911298835229,6.71089252375131));
#7304=CARTESIAN_POINT('Ctrl Pts',(0.369319867823668,0.784090370590367,6.74842072124706));
#7305=CARTESIAN_POINT('Ctrl Pts',(-0.137507651352654,0.841177037621035,
6.78200064499767));
#7306=CARTESIAN_POINT('Ctrl Pts',(-0.529655686323561,0.651783755111279,
6.81154496618753));
#7307=CARTESIAN_POINT('Ctrl Pts',(-0.763440172149879,0.359289385813127,
6.83697845361481));
#7308=CARTESIAN_POINT('Ctrl Pts',(-0.847211586055085,-0.0075813723717918,
6.86252259094478));
#7309=CARTESIAN_POINT('Ctrl Pts',(-0.763337400290734,-0.37595112739322,
6.88817526440515));
#7310=CARTESIAN_POINT('Ctrl Pts',(-0.526914388323573,-0.672730225787424,
6.91393691075106));
#7311=CARTESIAN_POINT('Ctrl Pts',(-0.183698562689997,-0.838276618909781,
6.93980597887144));
#7312=CARTESIAN_POINT('Ctrl Pts',(0.198889088741007,-0.838335964394735,
6.96578323697683));
#7313=CARTESIAN_POINT('Ctrl Pts',(0.545106947003364,-0.67180754918665,6.99186582148597));
#7314=CARTESIAN_POINT('Ctrl Pts',(0.785703595073577,-0.370406649743822,
7.01805361583897));
#7315=CARTESIAN_POINT('Ctrl Pts',(0.872119316826772,0.00721196141493378,
7.04434542939925));
#7316=CARTESIAN_POINT('Ctrl Pts',(0.785618184490446,0.386004597261683,7.07073989965295));
#7317=CARTESIAN_POINT('Ctrl Pts',(0.502331801959327,0.742799085163601,7.10165209474801));
#7318=CARTESIAN_POINT('Ctrl Pts',(-0.00621863503242753,0.921910367253639,
7.13714527690347));
#7319=CARTESIAN_POINT('Ctrl Pts',(-0.582851103775203,0.720649175322028,
7.17729562502998));
#7320=CARTESIAN_POINT('Ctrl Pts',(-0.909668842554882,0.201440782148561,
7.21765904401918));
#7321=CARTESIAN_POINT('Ctrl Pts',(-0.841213659251149,-0.41162272843365,
7.25823121418976));
#7322=CARTESIAN_POINT('Ctrl Pts',(-0.403262459624705,-0.850227454077078,
7.29900198947476));
#7323=CARTESIAN_POINT('Ctrl Pts',(0.215483513378321,-0.920627886099326,
7.33997190269741));
#7324=CARTESIAN_POINT('Ctrl Pts',(0.745429336505933,-0.587899220267355,
7.3811170115228));
#7325=CARTESIAN_POINT('Ctrl Pts',(0.883871797949062,-0.193227595737394,
7.40868621059601));
#7326=CARTESIAN_POINT('Ctrl Pts',(0.8838985919702,0.0053707753556189,7.42247342039135));
#7327=CARTESIAN_POINT('Ctrl Pts',(0.750293052325257,-0.00715957249020984,
5.50303372536175));
#7328=CARTESIAN_POINT('Ctrl Pts',(0.750270265731315,0.161735352510056,5.51475884548619));
#7329=CARTESIAN_POINT('Ctrl Pts',(0.632695708259348,0.496355890433882,5.53813632129441));
#7330=CARTESIAN_POINT('Ctrl Pts',(0.18381648383294,0.778081359279531,5.57298649818651));
#7331=CARTESIAN_POINT('Ctrl Pts',(-0.339280552431234,0.718378415257623,
5.6076202896276));
#7332=CARTESIAN_POINT('Ctrl Pts',(-0.709001801655557,0.347985187059841,
5.64204689091912));
#7333=CARTESIAN_POINT('Ctrl Pts',(-0.766698885918436,-0.16919180614749,
5.67627188750895));
#7334=CARTESIAN_POINT('Ctrl Pts',(-0.491102255096102,-0.606944769908898,
5.71030250431352));
#7335=CARTESIAN_POINT('Ctrl Pts',(-0.00508600093609879,-0.776552326514125,
5.74414714312887));
#7336=CARTESIAN_POINT('Ctrl Pts',(0.388081485630343,-0.638236893263609,
5.77157703947433));
#7337=CARTESIAN_POINT('Ctrl Pts',(0.596158844376195,-0.412773207290159,
5.79269814069561));
#7338=CARTESIAN_POINT('Ctrl Pts',(0.721744080724043,-0.15346691557969,5.81253217830301));
#7339=CARTESIAN_POINT('Ctrl Pts',(0.721291797138653,0.217701679185308,5.83724463136508));
#7340=CARTESIAN_POINT('Ctrl Pts',(0.492248297398938,0.553560023202817,5.86431639993153));
#7341=CARTESIAN_POINT('Ctrl Pts',(0.166319730891556,0.709798906698298,5.88884215604732));
#7342=CARTESIAN_POINT('Ctrl Pts',(-0.157783238149665,0.709878237357754,
5.9108529793775));
#7343=CARTESIAN_POINT('Ctrl Pts',(-0.449076273551193,0.569337590676698,
5.9328067996584));
#7344=CARTESIAN_POINT('Ctrl Pts',(-0.650064161571041,0.317172677340155,
5.95470251296732));
#7345=CARTESIAN_POINT('Ctrl Pts',(-0.721621885005776,0.00344024431033504,
5.97654562679051));
#7346=CARTESIAN_POINT('Ctrl Pts',(-0.661964542748072,-0.257286466758943,
5.99470556888389));
#7347=CARTESIAN_POINT('Ctrl Pts',(-0.550269179200512,-0.434720760832016,
6.00921182085571));
#7348=CARTESIAN_POINT('Ctrl Pts',(-0.402276742496014,-0.58292974874922,
6.02370295744568));
#7349=CARTESIAN_POINT('Ctrl Pts',(-0.162278225783224,-0.698511519651894,
6.04178723904388));
#7350=CARTESIAN_POINT('Ctrl Pts',(0.15678598762643,-0.698434753182134,6.06344900909546));
#7351=CARTESIAN_POINT('Ctrl Pts',(0.443832361536606,-0.560174670954122,
6.0850728430943));
#7352=CARTESIAN_POINT('Ctrl Pts',(0.641886657484862,-0.311548705127534,
6.10666325451466));
#7353=CARTESIAN_POINT('Ctrl Pts',(0.720903708581916,0.0325797868375459,
6.13061738623125));
#7354=CARTESIAN_POINT('Ctrl Pts',(0.604189885592221,0.409985700434759,6.15692940855218));
#7355=CARTESIAN_POINT('Ctrl Pts',(0.267732283871283,0.678698793729311,6.1855932204343));
#7356=CARTESIAN_POINT('Ctrl Pts',(-0.161176377088454,0.710602415331958,
6.2142207026778));
#7357=CARTESIAN_POINT('Ctrl Pts',(-0.53324499976805,0.49569736156826,6.2428252689349));
#7358=CARTESIAN_POINT('Ctrl Pts',(-0.71970802918005,0.108916638193807,6.27141553040571));
#7359=CARTESIAN_POINT('Ctrl Pts',(-0.653459538269235,-0.333490314335375,
6.30118792123758));
#7360=CARTESIAN_POINT('Ctrl Pts',(-0.320608653043408,-0.666665722932101,
6.33214798295712));
#7361=CARTESIAN_POINT('Ctrl Pts',(0.11110066391128,-0.714779997862643,6.36073732994674));
#7362=CARTESIAN_POINT('Ctrl Pts',(0.443426222920022,-0.554309028733026,
6.38577168766062));
#7363=CARTESIAN_POINT('Ctrl Pts',(0.640332263629123,-0.307185736963075,
6.4072429033775));
#7364=CARTESIAN_POINT('Ctrl Pts',(0.723203970884255,0.0529817392810816,
6.43231277693535));
#7365=CARTESIAN_POINT('Ctrl Pts',(0.579875213873492,0.464421357446747,6.46099511352603));
#7366=CARTESIAN_POINT('Ctrl Pts',(0.163540281833546,0.726164737539782,6.49332268601409));
#7367=CARTESIAN_POINT('Ctrl Pts',(-0.325806422280217,0.671154653749907,
6.52571901232898));
#7368=CARTESIAN_POINT('Ctrl Pts',(-0.675167952131389,0.322177709778464,
6.55819617950246));
#7369=CARTESIAN_POINT('Ctrl Pts',(-0.730838200739421,-0.169856078141101,
6.59076464701581));
#7370=CARTESIAN_POINT('Ctrl Pts',(-0.466820433339978,-0.590588090246883,
6.62343536526493));
#7371=CARTESIAN_POINT('Ctrl Pts',(0.00350996735505748,-0.755486408003205,
6.65621873257887));
#7372=CARTESIAN_POINT('Ctrl Pts',(0.475826092423244,-0.590582675084604,
6.6891250935537));
#7373=CARTESIAN_POINT('Ctrl Pts',(0.743223728972327,-0.165383236018042,
6.72216417731904));
#7374=CARTESIAN_POINT('Ctrl Pts',(0.687732640812107,0.335833673405217,6.75534872287688));
#7375=CARTESIAN_POINT('Ctrl Pts',(0.329161852114402,0.69473766380513,6.78868194987952));
#7376=CARTESIAN_POINT('Ctrl Pts',(-0.120255207878517,0.745235334942848,
6.81845529502086));
#7377=CARTESIAN_POINT('Ctrl Pts',(-0.467524502978826,0.57746640430216,6.84461903462784));
#7378=CARTESIAN_POINT('Ctrl Pts',(-0.674360922287096,0.318638588168112,
6.86712201294724));
#7379=CARTESIAN_POINT('Ctrl Pts',(-0.748404023106268,-0.00575219575844088,
6.88970750051041));
#7380=CARTESIAN_POINT('Ctrl Pts',(-0.674269101945005,-0.331252076513231,
6.91237414913092));
#7381=CARTESIAN_POINT('Ctrl Pts',(-0.465442485762675,-0.593360030871918,
6.93512642552479));
#7382=CARTESIAN_POINT('Ctrl Pts',(-0.162413298418938,-0.73950734230565,
6.95796516185281));
#7383=CARTESIAN_POINT('Ctrl Pts',(0.175299902719076,-0.739551441572441,
6.98089514210305));
#7384=CARTESIAN_POINT('Ctrl Pts',(0.48087309657339,-0.592568368954699,7.00391530912488));
#7385=CARTESIAN_POINT('Ctrl Pts',(0.693231099227059,-0.326542805878524,
7.02702898588934));
#7386=CARTESIAN_POINT('Ctrl Pts',(0.769520632376555,0.00680181224901938,
7.05023795575404));
#7387=CARTESIAN_POINT('Ctrl Pts',(0.693149586424791,0.341276467608696,7.07354385445611));
#7388=CARTESIAN_POINT('Ctrl Pts',(0.442928349106893,0.656453792431941,7.1008495131406));
#7389=CARTESIAN_POINT('Ctrl Pts',(-0.00655006027916784,0.814828143116751,
7.13222145322597));
#7390=CARTESIAN_POINT('Ctrl Pts',(-0.51677651805262,0.636849892039306,7.16774598353412));
#7391=CARTESIAN_POINT('Ctrl Pts',(-0.806409087124653,0.176948274600164,
7.20350474142154));
#7392=CARTESIAN_POINT('Ctrl Pts',(-0.745817965655065,-0.367012141382838,
7.2395023580954));
#7393=CARTESIAN_POINT('Ctrl Pts',(-0.356682875026977,-0.756951656680894,
7.27574101303561));
#7394=CARTESIAN_POINT('Ctrl Pts',(0.194324484528691,-0.819874060139303,
7.3122257656988));
#7395=CARTESIAN_POINT('Ctrl Pts',(0.667449116817723,-0.523027248491166,
7.34895409901446));
#7396=CARTESIAN_POINT('Ctrl Pts',(0.791458463792618,-0.170101188152833,
7.37361186684348));
#7397=CARTESIAN_POINT('Ctrl Pts',(0.791482481276893,0.00791737913227817,
7.38597037371902));
#7398=CARTESIAN_POINT('Ctrl Pts',(0.849598076317196,-0.00712734349710777,
5.50276247098815));
#7399=CARTESIAN_POINT('Ctrl Pts',(0.849572315215897,0.183814720194332,5.51601816019011));
#7400=CARTESIAN_POINT('Ctrl Pts',(0.716484451910036,0.562864504493882,5.5424997573337));
#7401=CARTESIAN_POINT('Ctrl Pts',(0.20809212706776,0.881898014322701,5.58196713633214));
#7402=CARTESIAN_POINT('Ctrl Pts',(-0.384533142466098,0.814321092392168,
5.6212091202806));
#7403=CARTESIAN_POINT('Ctrl Pts',(-0.803342488001547,0.394693505033448,
5.66020880663821));
#7404=CARTESIAN_POINT('Ctrl Pts',(-0.868627634713463,-0.190973266163329,
5.69896909964657));
#7405=CARTESIAN_POINT('Ctrl Pts',(-0.556653040774226,-0.686349150395686,
5.7374846668518));
#7406=CARTESIAN_POINT('Ctrl Pts',(-0.00707997145394115,-0.878014145711534,
5.77575459287924));
#7407=CARTESIAN_POINT('Ctrl Pts',(0.436900544149483,-0.72169954588876,5.80673549990624));
#7408=CARTESIAN_POINT('Ctrl Pts',(0.671606542222444,-0.467350263792894,
5.83056225412086));
#7409=CARTESIAN_POINT('Ctrl Pts',(0.813155385970533,-0.1750292179711,5.85292188205288));
#7410=CARTESIAN_POINT('Ctrl Pts',(0.812540057938428,0.242883178054026,5.88074814557167));
#7411=CARTESIAN_POINT('Ctrl Pts',(0.554998700939117,0.6202772367454,5.91117655608676));
#7412=CARTESIAN_POINT('Ctrl Pts',(0.189304493774159,0.795493011487289,5.93869516979536));
#7413=CARTESIAN_POINT('Ctrl Pts',(-0.173712239990491,0.795504865118224,
5.96335163063203));
#7414=CARTESIAN_POINT('Ctrl Pts',(-0.499345414071431,0.638313353697133,
5.98789731654311));
#7415=CARTESIAN_POINT('Ctrl Pts',(-0.72356068389146,0.356867037202337,6.01233388291633));
#7416=CARTESIAN_POINT('Ctrl Pts',(-0.803163168357719,0.00747357176146625,
6.03666105392709));
#7417=CARTESIAN_POINT('Ctrl Pts',(-0.736797982336716,-0.28222992698738,
6.05684360012597));
#7418=CARTESIAN_POINT('Ctrl Pts',(-0.612891815719577,-0.479031268493863,
6.07293511022899));
#7419=CARTESIAN_POINT('Ctrl Pts',(-0.448917230819194,-0.643222296978376,
6.08899082487842));
#7420=CARTESIAN_POINT('Ctrl Pts',(-0.18345184155449,-0.770972157981274,
6.10899459772628));
#7421=CARTESIAN_POINT('Ctrl Pts',(0.168509519247147,-0.770779631725406,
6.1328926650123));
#7422=CARTESIAN_POINT('Ctrl Pts',(0.484258307101598,-0.618569501699951,
6.15668614964677));
#7423=CARTESIAN_POINT('Ctrl Pts',(0.7014559478794,-0.345739709198507,6.18037560572192));
#7424=CARTESIAN_POINT('Ctrl Pts',(0.787759201210554,0.0307483449030446,
6.20658402952268));
#7425=CARTESIAN_POINT('Ctrl Pts',(0.660297100374137,0.44205148705441,6.23526827245269));
#7426=CARTESIAN_POINT('Ctrl Pts',(0.29489586174265,0.733477282971818,6.2663838499292));
#7427=CARTESIAN_POINT('Ctrl Pts',(-0.168647261234911,0.767641847640704,
6.2973293246475));
#7428=CARTESIAN_POINT('Ctrl Pts',(-0.568727882191308,0.536181820843462,
6.32810567535681));
#7429=CARTESIAN_POINT('Ctrl Pts',(-0.768048251626985,0.121961889290114,
6.35871685457357));
#7430=CARTESIAN_POINT('Ctrl Pts',(-0.697107833504566,-0.349296397819721,
6.39043824166099));
#7431=CARTESIAN_POINT('Ctrl Pts',(-0.344045555812211,-0.701995892428354,
6.42325363059534));
#7432=CARTESIAN_POINT('Ctrl Pts',(0.110773521189623,-0.752235352072163,
6.45337778122228));
#7433=CARTESIAN_POINT('Ctrl Pts',(0.458965638454581,-0.583886825258837,
6.47961716649731));
#7434=CARTESIAN_POINT('Ctrl Pts',(0.664381883487217,-0.325864755846388,
6.50203114286227));
#7435=CARTESIAN_POINT('Ctrl Pts',(0.750332653299937,0.0485776788759206,
6.52809351690923));
#7436=CARTESIAN_POINT('Ctrl Pts',(0.601674226486008,0.473897649396157,6.55776163974272));
#7437=CARTESIAN_POINT('Ctrl Pts',(0.173613673117217,0.742348086642931,6.59098287751551));
#7438=CARTESIAN_POINT('Ctrl Pts',(-0.3258350440189,0.685649541287933,6.62406030334558));
#7439=CARTESIAN_POINT('Ctrl Pts',(-0.679731238547397,0.331354382468774,
6.65700275666622));
#7440=CARTESIAN_POINT('Ctrl Pts',(-0.735255898447251,-0.164397347346024,
6.6898206739066));
#7441=CARTESIAN_POINT('Ctrl Pts',(-0.470558029977308,-0.585159244984441,
6.7225241569716));
#7442=CARTESIAN_POINT('Ctrl Pts',(-0.00278192751448173,-0.748569972495831,
6.75512382817215));
#7443=CARTESIAN_POINT('Ctrl Pts',(0.46350519113553,-0.58518407843876,6.78763042208935));
#7444=CARTESIAN_POINT('Ctrl Pts',(0.725410474458316,-0.167706567477984,
6.82005514647598));
#7445=CARTESIAN_POINT('Ctrl Pts',(0.670774587918448,0.320804047707368,6.85240545447397));
#7446=CARTESIAN_POINT('Ctrl Pts',(0.323092957157568,0.668041717311718,6.88470045447928));
#7447=CARTESIAN_POINT('Ctrl Pts',(-0.109494451463983,0.716184576245998,
6.91336373465137));
#7448=CARTESIAN_POINT('Ctrl Pts',(-0.44188826662967,0.555407233522295,6.93841735921765));
#7449=CARTESIAN_POINT('Ctrl Pts',(-0.639012403336459,0.308500858246645,
6.95988071793453));
#7450=CARTESIAN_POINT('Ctrl Pts',(-0.709192507424316,0.00040641570270789,
6.98133136104379));
#7451=CARTESIAN_POINT('Ctrl Pts',(-0.638918625948615,-0.307487189319304,
7.00277862675193));
#7452=CARTESIAN_POINT('Ctrl Pts',(-0.442028652642433,-0.554399048208452,
7.02422233485342));
#7453=CARTESIAN_POINT('Ctrl Pts',(-0.157482946544586,-0.691481626684627,
7.0456683320825));
#7454=CARTESIAN_POINT('Ctrl Pts',(0.15835851542768,-0.691398914091788,7.06711532573104));
#7455=CARTESIAN_POINT('Ctrl Pts',(0.44307547960184,-0.554307235545146,7.08857226527194));
#7456=CARTESIAN_POINT('Ctrl Pts',(0.64018584092255,-0.307192493791569,7.11004002498397));
#7457=CARTESIAN_POINT('Ctrl Pts',(0.71067332605218,0.00132671397574847,
7.13152214083118));
#7458=CARTESIAN_POINT('Ctrl Pts',(0.640127181409651,0.309809306958141,7.15302225181439));
#7459=CARTESIAN_POINT('Ctrl Pts',(0.409965562319378,0.59950154513597,7.1781297331652));
#7460=CARTESIAN_POINT('Ctrl Pts',(-0.00180430761257666,0.744250295435473,
7.20686838534354));
#7461=CARTESIAN_POINT('Ctrl Pts',(-0.46689999412445,0.581628177637233,7.23926440850474));
#7462=CARTESIAN_POINT('Ctrl Pts',(-0.729602505011613,0.163869023223047,
7.27173917712393));
#7463=CARTESIAN_POINT('Ctrl Pts',(-0.674485616164893,-0.328104186907804,
7.3043020520652));
#7464=CARTESIAN_POINT('Ctrl Pts',(-0.32358572160231,-0.679299557613987,
7.33696613118188));
#7465=CARTESIAN_POINT('Ctrl Pts',(0.171370920939519,-0.735610678055291,
7.36973771478191));
#7466=CARTESIAN_POINT('Ctrl Pts',(0.594929256360531,-0.469509634858928,
7.40263639340595));
#7467=CARTESIAN_POINT('Ctrl Pts',(0.705563583847616,-0.154509464242322,
7.42464584593578));
#7468=CARTESIAN_POINT('Ctrl Pts',(0.705585033709163,0.00447777927316105,
7.4356831493591));
#7469=CARTESIAN_POINT('Ctrl Pts',(0.911787311372316,-0.00175313599507732,
5.42547035947661));
#7470=CARTESIAN_POINT('Ctrl Pts',(0.911759679946333,0.203051830949188,5.43968844708048));
#7471=CARTESIAN_POINT('Ctrl Pts',(0.768907437119982,0.61071591344494,5.46816718430648));
#7472=CARTESIAN_POINT('Ctrl Pts',(0.220284165601068,0.955502366817236,5.51077805671262));
#7473=CARTESIAN_POINT('Ctrl Pts',(-0.422243656323184,0.882710139668278,
5.55332558349325));
#7474=CARTESIAN_POINT('Ctrl Pts',(-0.878386039542625,0.426289581625414,
5.5957765844892));
#7475=CARTESIAN_POINT('Ctrl Pts',(-0.950141006447777,-0.213553723589873,
5.63813025439539));
#7476=CARTESIAN_POINT('Ctrl Pts',(-0.60835728725253,-0.757014115469509,
5.68037224924266));
#7477=CARTESIAN_POINT('Ctrl Pts',(-0.00366338310403281,-0.968314430281517,
5.72249300107482));
#7478=CARTESIAN_POINT('Ctrl Pts',(0.486718248881734,-0.795970516833383,
5.75670865791863));
#7479=CARTESIAN_POINT('Ctrl Pts',(0.74653021351722,-0.514477549037207,5.78308078863264));
#7480=CARTESIAN_POINT('Ctrl Pts',(0.903446118847398,-0.190511009717507,
5.80786424281498));
#7481=CARTESIAN_POINT('Ctrl Pts',(0.90295145376886,0.273634535370419,5.8387700025228));
#7482=CARTESIAN_POINT('Ctrl Pts',(0.616343546706946,0.693954207986666,5.87265196790731));
#7483=CARTESIAN_POINT('Ctrl Pts',(0.208328450290096,0.889559871552857,5.90335942490417));
#7484=CARTESIAN_POINT('Ctrl Pts',(-0.197431208021256,0.889652469467467,
5.93091996947637));
#7485=CARTESIAN_POINT('Ctrl Pts',(-0.562029250439909,0.713737268348937,
5.95840063131195));
#7486=CARTESIAN_POINT('Ctrl Pts',(-0.813494233574056,0.39820149627948,5.98580131723829));
#7487=CARTESIAN_POINT('Ctrl Pts',(-0.902946074851847,0.0058870464447316,
6.01311843029465));
#7488=CARTESIAN_POINT('Ctrl Pts',(-0.828377509677636,-0.319866751453087,
6.03581174060078));
#7489=CARTESIAN_POINT('Ctrl Pts',(-0.688936970150508,-0.541360820821501,
6.05392170180393));
#7490=CARTESIAN_POINT('Ctrl Pts',(-0.504293132651573,-0.726263454623667,
6.07200206864918));
#7491=CARTESIAN_POINT('Ctrl Pts',(-0.205118119105362,-0.870286210128437,
6.0945471479209));
#7492=CARTESIAN_POINT('Ctrl Pts',(0.191971983732839,-0.870117700265186,
6.12150897978661));
#7493=CARTESIAN_POINT('Ctrl Pts',(0.548553466642107,-0.698273117288175,
6.14837718076188));
#7494=CARTESIAN_POINT('Ctrl Pts',(0.794052616995502,-0.389950825708538,
6.17514969693223));
#7495=CARTESIAN_POINT('Ctrl Pts',(0.891698024550524,0.0358312226908213,
6.20478886300642));
#7496=CARTESIAN_POINT('Ctrl Pts',(0.74749095040922,0.501334011480795,6.23725086378811));
#7497=CARTESIAN_POINT('Ctrl Pts',(0.333743343393983,0.831378563455359,6.27248425191807));
#7498=CARTESIAN_POINT('Ctrl Pts',(-0.19134387466354,0.870105625426578,6.3075348767601));
#7499=CARTESIAN_POINT('Ctrl Pts',(-0.644616547373273,0.607881105022717,
6.34239973374175));
#7500=CARTESIAN_POINT('Ctrl Pts',(-0.870417110421222,0.138612855199806,
6.37707657725051));
#7501=CARTESIAN_POINT('Ctrl Pts',(-0.790048775469081,-0.39510788351932,
6.41299953612703));
#7502=CARTESIAN_POINT('Ctrl Pts',(-0.390383204661376,-0.794274173322802,
6.45013660062964));
#7503=CARTESIAN_POINT('Ctrl Pts',(0.123964069137483,-0.851002982786416,
6.48419818277685));
#7504=CARTESIAN_POINT('Ctrl Pts',(0.517349958215306,-0.660759929294058,
6.51384272570464));
#7505=CARTESIAN_POINT('Ctrl Pts',(0.749191592206741,-0.369479150376496,
6.53914157276564));
#7506=CARTESIAN_POINT('Ctrl Pts',(0.846067098454331,0.052769037404062,6.56852738290555));
#7507=CARTESIAN_POINT('Ctrl Pts',(0.678541487051601,0.531594017531224,6.60192411587722));
#7508=CARTESIAN_POINT('Ctrl Pts',(0.197445708687755,0.833056774682923,6.63924640568331));
#7509=CARTESIAN_POINT('Ctrl Pts',(-0.362407034535075,0.76926077023711,6.67631865996902));
#7510=CARTESIAN_POINT('Ctrl Pts',(-0.757891257853047,0.372960662447378,
6.7131423125874));
#7511=CARTESIAN_POINT('Ctrl Pts',(-0.819502812158925,-0.17971389368945,
6.74971854734871));
#7512=CARTESIAN_POINT('Ctrl Pts',(-0.525117958852971,-0.647082052916212,
6.78604945080241));
#7513=CARTESIAN_POINT('Ctrl Pts',(-0.00706009915885147,-0.827706145589558,
6.82213749402266));
#7514=CARTESIAN_POINT('Ctrl Pts',(0.507168732938518,-0.647142083318005,
6.85798569667506));
#7515=CARTESIAN_POINT('Ctrl Pts',(0.794559460318739,-0.188312585352296,
6.89359746949419));
#7516=CARTESIAN_POINT('Ctrl Pts',(0.734412407851191,0.346047384757273,6.92898046138837));
#7517=CARTESIAN_POINT('Ctrl Pts',(0.35554627917015,0.723799648271606,6.96413145325235));
#7518=CARTESIAN_POINT('Ctrl Pts',(-0.113206435891536,0.775602232806529,
6.99517934888198));
#7519=CARTESIAN_POINT('Ctrl Pts',(-0.471799040782441,0.601968214167806,
7.0222090326148));
#7520=CARTESIAN_POINT('Ctrl Pts',(-0.6836661147338,0.336404243341276,7.04528069450069));
#7521=CARTESIAN_POINT('Ctrl Pts',(-0.758726003996092,0.0062400461075705,
7.06826344122686));
#7522=CARTESIAN_POINT('Ctrl Pts',(-0.6835849590214,-0.322409867084328,7.09115224380289));
#7523=CARTESIAN_POINT('Ctrl Pts',(-0.474072442185209,-0.584919976115439,
7.11395355010067));
#7524=CARTESIAN_POINT('Ctrl Pts',(-0.172560181698569,-0.730020088066619,
7.13666650878931));
#7525=CARTESIAN_POINT('Ctrl Pts',(0.16078217307758,-0.729778328929261,7.15929927954856));
#7526=CARTESIAN_POINT('Ctrl Pts',(0.459989212508115,-0.585545816121325,
7.18184723354721));
#7527=CARTESIAN_POINT('Ctrl Pts',(0.666223161118391,-0.32674631555655,7.20431603435277));
#7528=CARTESIAN_POINT('Ctrl Pts',(0.739554158501798,-0.00504686561265504,
7.22670799379599));
#7529=CARTESIAN_POINT('Ctrl Pts',(0.666159558065311,0.315205418031567,7.24902537021377));
#7530=CARTESIAN_POINT('Ctrl Pts',(0.428020561210259,0.614621005636118,7.27497954766194));
#7531=CARTESIAN_POINT('Ctrl Pts',(0.00440289337514439,0.763018006049135,
7.30452179484735));
#7532=CARTESIAN_POINT('Ctrl Pts',(-0.470624128322024,0.596319364034835,
7.33761244678054));
#7533=CARTESIAN_POINT('Ctrl Pts',(-0.736811683564632,0.171965979607826,
7.37056624676418));
#7534=CARTESIAN_POINT('Ctrl Pts',(-0.68068387352667,-0.324086643305756,
7.4033919913947));
#7535=CARTESIAN_POINT('Ctrl Pts',(-0.328791217341046,-0.675487864461335,
7.43610391008164));
#7536=CARTESIAN_POINT('Ctrl Pts',(0.163774412047771,-0.731012482418632,
7.4687018632077));
#7537=CARTESIAN_POINT('Ctrl Pts',(0.582152961317522,-0.467440680790944,
7.50121977146286));
#7538=CARTESIAN_POINT('Ctrl Pts',(0.690380552641563,-0.158133439986746,
7.52281364669809));
#7539=CARTESIAN_POINT('Ctrl Pts',(0.690401574315868,-0.00231993767140268,
7.53363062084317));
#7540=CARTESIAN_POINT('Ctrl Pts',(0.889359432826132,0.00495444760725769,
5.32880713791624));
#7541=CARTESIAN_POINT('Ctrl Pts',(0.889332447864276,0.204967802847453,5.34269257951066));
#7542=CARTESIAN_POINT('Ctrl Pts',(0.750004347575518,0.603672713614473,5.37053043303203));
#7543=CARTESIAN_POINT('Ctrl Pts',(0.21096706922133,0.94314460394843,5.41241969183905));
#7544=CARTESIAN_POINT('Ctrl Pts',(-0.423963274156834,0.87171349864309,5.45445132266662));
#7545=CARTESIAN_POINT('Ctrl Pts',(-0.877374490363263,0.418799407840054,
5.4966071161887));
#7546=CARTESIAN_POINT('Ctrl Pts',(-0.949545774103564,-0.219892556824646,
5.53888079270843));
#7547=CARTESIAN_POINT('Ctrl Pts',(-0.607068575689537,-0.765494054358749,
5.58125986451715));
#7548=CARTESIAN_POINT('Ctrl Pts',(0.00261167844658479,-0.97913119777945,
5.62373519298684));
#7549=CARTESIAN_POINT('Ctrl Pts',(0.499852533620251,-0.8048463257254,5.65841239967706));
#7550=CARTESIAN_POINT('Ctrl Pts',(0.764265215589788,-0.518466038803169,
5.68524380080038));
#7551=CARTESIAN_POINT('Ctrl Pts',(0.924328881255501,-0.188150671604858,
5.71051448038525));
#7552=CARTESIAN_POINT('Ctrl Pts',(0.924132430512447,0.286757902074732,5.74213409224145));
#7553=CARTESIAN_POINT('Ctrl Pts',(0.62986087869606,0.718937325916808,5.77695468815655));
#7554=CARTESIAN_POINT('Ctrl Pts',(0.208953775300158,0.920912997464213,5.80863418802737));
#7555=CARTESIAN_POINT('Ctrl Pts',(-0.211068988110463,0.921157282542793,
5.83716174516452));
#7556=CARTESIAN_POINT('Ctrl Pts',(-0.589810577699277,0.738585626106938,
5.86570218738055));
#7557=CARTESIAN_POINT('Ctrl Pts',(-0.85194552766839,0.409898301969846,5.89425134138179));
#7558=CARTESIAN_POINT('Ctrl Pts',(-0.945597945878367,-0.000176678256206242,
5.92280607763768));
#7559=CARTESIAN_POINT('Ctrl Pts',(-0.867511729419428,-0.341824865852328,
5.94660339370044));
#7560=CARTESIAN_POINT('Ctrl Pts',(-0.720944780593085,-0.574681060925877,
5.96564071682787));
#7561=CARTESIAN_POINT('Ctrl Pts',(-0.526555141270467,-0.769375552079073,
5.98467700523746));
#7562=CARTESIAN_POINT('Ctrl Pts',(-0.210870756052851,-0.921475670946048,
6.00846936790163));
#7563=CARTESIAN_POINT('Ctrl Pts',(0.209506448294534,-0.921438779399368,
6.03701193615958));
#7564=CARTESIAN_POINT('Ctrl Pts',(0.588220824730041,-0.739083885420811,
6.0655428661009));
#7565=CARTESIAN_POINT('Ctrl Pts',(0.849810718286318,-0.410765395052392,
6.09405857275419));
#7566=CARTESIAN_POINT('Ctrl Pts',(0.95427567990068,0.0440511715684175,6.12572236137368));
#7567=CARTESIAN_POINT('Ctrl Pts',(0.799967960952214,0.54314825140328,6.16052078866217));
#7568=CARTESIAN_POINT('Ctrl Pts',(0.354946991113063,0.898546473402006,6.19843574858538));
#7569=CARTESIAN_POINT('Ctrl Pts',(-0.212199085766547,0.940684954588202,
6.23629684514792));
#7570=CARTESIAN_POINT('Ctrl Pts',(-0.703732454340991,0.656671161576527,
6.27409476897982));
#7571=CARTESIAN_POINT('Ctrl Pts',(-0.949639640621547,0.146281182681,6.31182133692065));
#7572=CARTESIAN_POINT('Ctrl Pts',(-0.862200374710721,-0.436390813484725,
6.35103882924841));
#7573=CARTESIAN_POINT('Ctrl Pts',(-0.424615550503731,-0.87396308504598,
6.39172839424829));
#7574=CARTESIAN_POINT('Ctrl Pts',(0.140875049279472,-0.936660006455991,
6.42918239638723));
#7575=CARTESIAN_POINT('Ctrl Pts',(0.574670287621894,-0.727011014446981,
6.46186903203473));
#7576=CARTESIAN_POINT('Ctrl Pts',(0.83093266790137,-0.405200393190354,6.48982632103455));
#7577=CARTESIAN_POINT('Ctrl Pts',(0.938317766588939,0.0623494789078903,
6.52236975513327));
#7578=CARTESIAN_POINT('Ctrl Pts',(0.752579540678534,0.594055251251905,6.55945509994811));
#7579=CARTESIAN_POINT('Ctrl Pts',(0.217059284541729,0.929973502219806,6.60101727981861));
#7580=CARTESIAN_POINT('Ctrl Pts',(-0.408026785252189,0.859019100893442,
6.6424136299843));
#7581=CARTESIAN_POINT('Ctrl Pts',(-0.850845977716372,0.415638179906151,
6.68363494790014));
#7582=CARTESIAN_POINT('Ctrl Pts',(-0.920184777472661,-0.204329024249146,
6.72467349392044));
#7583=CARTESIAN_POINT('Ctrl Pts',(-0.589428074185655,-0.729814282912527,
6.76552142650441));
#7584=CARTESIAN_POINT('Ctrl Pts',(-0.00604978450581677,-0.933394312826398,
6.80617154371966));
#7585=CARTESIAN_POINT('Ctrl Pts',(0.57404869025302,-0.72985742835735,6.84661700406497));
#7586=CARTESIAN_POINT('Ctrl Pts',(0.898783211561984,-0.211649435517353,
6.8868516259356));
#7587=CARTESIAN_POINT('Ctrl Pts',(0.830853561486015,0.392570978289185,6.92686564614092));
#7588=CARTESIAN_POINT('Ctrl Pts',(0.402102843122056,0.820171632165624,6.96666187541315));
#7589=CARTESIAN_POINT('Ctrl Pts',(-0.128752136760593,0.87885181573823,7.0018337119622));
#7590=CARTESIAN_POINT('Ctrl Pts',(-0.534933891924655,0.682185839564183,
7.03245541763881));
#7591=CARTESIAN_POINT('Ctrl Pts',(-0.774943785493673,0.381327511531892,
7.05860032562784));
#7592=CARTESIAN_POINT('Ctrl Pts',(-0.859966110515312,0.00734177845082202,
7.08463607645075));
#7593=CARTESIAN_POINT('Ctrl Pts',(-0.774831422913684,-0.364904312674865,
7.11056853328824));
#7594=CARTESIAN_POINT('Ctrl Pts',(-0.537583138232402,-0.662143756003773,
7.13639250543407));
#7595=CARTESIAN_POINT('Ctrl Pts',(-0.196279169025999,-0.826362279426242,
7.16211006197668));
#7596=CARTESIAN_POINT('Ctrl Pts',(0.180788904256726,-0.82607059745876,7.18771480491698));
#7597=CARTESIAN_POINT('Ctrl Pts',(0.519038634180724,-0.662978803853832,
7.21321277550856));
#7598=CARTESIAN_POINT('Ctrl Pts',(0.751978439186691,-0.370613914749894,
7.23860036966167));
#7599=CARTESIAN_POINT('Ctrl Pts',(0.834701683971329,-0.00754650688657486,
7.26387733624003));
#7600=CARTESIAN_POINT('Ctrl Pts',(0.751920252216622,0.353483451503403,7.28904368273798));
#7601=CARTESIAN_POINT('Ctrl Pts',(0.483730036422595,0.690590593695916,7.31827398545647));
#7602=CARTESIAN_POINT('Ctrl Pts',(0.00742785048027893,0.857265989116031,
7.35149921639049));
#7603=CARTESIAN_POINT('Ctrl Pts',(-0.525293231887737,0.670073438058683,
7.38862588821794));
#7604=CARTESIAN_POINT('Ctrl Pts',(-0.822869944746703,0.195197072733832,
7.42550481928346));
#7605=CARTESIAN_POINT('Ctrl Pts',(-0.759959606004209,-0.358130855720698,
7.46213543363099));
#7606=CARTESIAN_POINT('Ctrl Pts',(-0.368415214766548,-0.748693330694505,
7.49852208898732));
#7607=CARTESIAN_POINT('Ctrl Pts',(0.177541916017237,-0.809855769006471,
7.53466251134493));
#7608=CARTESIAN_POINT('Ctrl Pts',(0.639295990646259,-0.518615892317653,
7.57056942797824));
#7609=CARTESIAN_POINT('Ctrl Pts',(0.758201052838224,-0.178255309934477,
7.59433715581631));
#7610=CARTESIAN_POINT('Ctrl Pts',(0.758224108327783,-0.00736708650145173,
7.60620065587956));
#7611=CARTESIAN_POINT('Ctrl Pts',(0.829918995390605,0.00692962491070555,
5.30024010712383));
#7612=CARTESIAN_POINT('Ctrl Pts',(0.829893790259993,0.193750817013165,5.31320971482039));
#7613=CARTESIAN_POINT('Ctrl Pts',(0.699822285583035,0.566145381882556,5.3392101566049));
#7614=CARTESIAN_POINT('Ctrl Pts',(0.195323515234371,0.88416117171195,5.37842883489126));
#7615=CARTESIAN_POINT('Ctrl Pts',(-0.400343151138505,0.817346474568011,
5.41785865980122));
#7616=CARTESIAN_POINT('Ctrl Pts',(-0.826817727686594,0.391700174990477,
5.4574958434249));
#7617=CARTESIAN_POINT('Ctrl Pts',(-0.895091678603364,-0.210180305596499,
5.49733544534094));
#7618=CARTESIAN_POINT('Ctrl Pts',(-0.571783532988076,-0.72574941013594,
5.53737192540201));
#7619=CARTESIAN_POINT('Ctrl Pts',(0.00554627097635579,-0.928352383739425,
5.57760056939562));
#7620=CARTESIAN_POINT('Ctrl Pts',(0.477799679854192,-0.76307476144334,5.61052921806703));
#7621=CARTESIAN_POINT('Ctrl Pts',(0.729410852594162,-0.490616169914011,
5.63605789108779));
#7622=CARTESIAN_POINT('Ctrl Pts',(0.881919476817548,-0.175979128010471,
5.66013043243701));
#7623=CARTESIAN_POINT('Ctrl Pts',(0.881906152444497,0.277265930526209,5.69030700929344));
#7624=CARTESIAN_POINT('Ctrl Pts',(0.600514890488868,0.690886371812261,5.72362170442843));
#7625=CARTESIAN_POINT('Ctrl Pts',(0.196921477412404,0.884675277260858,5.75399952860311));
#7626=CARTESIAN_POINT('Ctrl Pts',(-0.206656190820974,0.885009407611865,
5.78140796402136));
#7627=CARTESIAN_POINT('Ctrl Pts',(-0.571352525906284,0.709312471916405,
5.80888598178339));
#7628=CARTESIAN_POINT('Ctrl Pts',(-0.824322784093117,0.39228222278969,5.8364255516956));
#7629=CARTESIAN_POINT('Ctrl Pts',(-0.914955919505048,-0.00412326864883124,
5.86402777825679));
#7630=CARTESIAN_POINT('Ctrl Pts',(-0.839394814319228,-0.335102288993869,
5.88707765903504));
#7631=CARTESIAN_POINT('Ctrl Pts',(-0.697194784237861,-0.561053925833896,
5.90554855730548));
#7632=CARTESIAN_POINT('Ctrl Pts',(-0.508394551716055,-0.75017609097147,
5.9240379575655));
#7633=CARTESIAN_POINT('Ctrl Pts',(-0.201331843767861,-0.89822223947356,
5.94717992736717));
#7634=CARTESIAN_POINT('Ctrl Pts',(0.208503775368862,-0.898293333883727,
5.97500361673599));
#7635=CARTESIAN_POINT('Ctrl Pts',(0.578566181754719,-0.72022509709185,6.00287494476189));
#7636=CARTESIAN_POINT('Ctrl Pts',(0.834785028018541,-0.398807815817064,
6.03079323532));
#7637=CARTESIAN_POINT('Ctrl Pts',(0.937421618538533,0.0474693145637866,
6.06185942553353));
#7638=CARTESIAN_POINT('Ctrl Pts',(0.785808706512713,0.53858289651246,6.09609235737173));
#7639=CARTESIAN_POINT('Ctrl Pts',(0.346833476768302,0.889498241929319,6.13350258691761));
#7640=CARTESIAN_POINT('Ctrl Pts',(-0.214450953963022,0.931459250732699,
6.17096335002368));
#7641=CARTESIAN_POINT('Ctrl Pts',(-0.702523232936964,0.649744126672763,
6.20847735887153));
#7642=CARTESIAN_POINT('Ctrl Pts',(-0.947620032703892,0.141637172177686,
6.24603852533507));
#7643=CARTESIAN_POINT('Ctrl Pts',(-0.860569087705711,-0.440346323520561,
6.28520072180747));
#7644=CARTESIAN_POINT('Ctrl Pts',(-0.422417509108382,-0.879011958721694,
6.32595508450303));
#7645=CARTESIAN_POINT('Ctrl Pts',(0.146053510149855,-0.942361769529175,
6.36359784749923));
#7646=CARTESIAN_POINT('Ctrl Pts',(0.583529811691089,-0.731092224974979,
6.39655251871174));
#7647=CARTESIAN_POINT('Ctrl Pts',(0.842579028174264,-0.405926837413371,
6.42480144817265));
#7648=CARTESIAN_POINT('Ctrl Pts',(0.951487177832284,0.0675991994034292,
6.45775864234018));
#7649=CARTESIAN_POINT('Ctrl Pts',(0.763141746082221,0.607725575505774,6.49541116932488));
#7650=CARTESIAN_POINT('Ctrl Pts',(0.217574487524898,0.950392778021499,6.53775763542001));
#7651=CARTESIAN_POINT('Ctrl Pts',(-0.42166740973873,0.878191572890031,6.58007504544765));
#7652=CARTESIAN_POINT('Ctrl Pts',(-0.876250398231941,0.423545215383675,
6.62235503675604));
#7653=CARTESIAN_POINT('Ctrl Pts',(-0.947987096499237,-0.21459643925478,
6.6645859298645));
#7654=CARTESIAN_POINT('Ctrl Pts',(-0.606705076713124,-0.757473932422971,
6.70675774894366));
#7655=CARTESIAN_POINT('Ctrl Pts',(-0.00241202776964925,-0.968727997454768,
6.74885991888449));
#7656=CARTESIAN_POINT('Ctrl Pts',(0.600624482148029,-0.757509613558942,
6.79088237303874));
#7657=CARTESIAN_POINT('Ctrl Pts',(0.939452177122731,-0.217421016410473,
6.8328144749144));
#7658=CARTESIAN_POINT('Ctrl Pts',(0.868758799747721,0.414536277515111,6.87465507197778));
#7659=CARTESIAN_POINT('Ctrl Pts',(0.419290549746345,0.863247184920627,6.91637647714826));
#7660=CARTESIAN_POINT('Ctrl Pts',(-0.139084650191804,0.925265402913614,
6.95335818017224));
#7661=CARTESIAN_POINT('Ctrl Pts',(-0.567454545740675,0.717965354424563,
6.98564100520883));
#7662=CARTESIAN_POINT('Ctrl Pts',(-0.821064769263926,0.400211556185252,
7.0132490098583));
#7663=CARTESIAN_POINT('Ctrl Pts',(-0.91112933929112,0.00438963293201363,
7.04080231652177));
#7664=CARTESIAN_POINT('Ctrl Pts',(-0.820966778853315,-0.390275853878312,
7.0682856755789));
#7665=CARTESIAN_POINT('Ctrl Pts',(-0.569057996064222,-0.706001271167066,
7.09570447796615));
#7666=CARTESIAN_POINT('Ctrl Pts',(-0.206027274734066,-0.880764451318613,
7.1230513221731));
#7667=CARTESIAN_POINT('Ctrl Pts',(0.195812674813625,-0.880515195886687,
7.15033395522949));
#7668=CARTESIAN_POINT('Ctrl Pts',(0.556847139748695,-0.706517914293179,
7.17753857633508));
#7669=CARTESIAN_POINT('Ctrl Pts',(0.805895709935206,-0.394032847218828,
7.20466842663578));
#7670=CARTESIAN_POINT('Ctrl Pts',(0.894511398596212,-0.00535918267020315,
7.2317212151674));
#7671=CARTESIAN_POINT('Ctrl Pts',(0.805810304168001,0.381721934163946,7.25869451527825));
#7672=CARTESIAN_POINT('Ctrl Pts',(0.517921324180488,0.743697104768732,7.29007024661223));
#7673=CARTESIAN_POINT('Ctrl Pts',(0.00578604455006559,0.923078227892816,
7.32578329054371));
#7674=CARTESIAN_POINT('Ctrl Pts',(-0.568243145767641,0.721567999099011,
7.3657709938243));
#7675=CARTESIAN_POINT('Ctrl Pts',(-0.889554950114489,0.209118291781916,
7.40555959496073));
#7676=CARTESIAN_POINT('Ctrl Pts',(-0.821710123582801,-0.38904286980981,
7.44514503289073));
#7677=CARTESIAN_POINT('Ctrl Pts',(-0.397947019918738,-0.811956407468429,
7.48452302388204));
#7678=CARTESIAN_POINT('Ctrl Pts',(0.193792979174468,-0.878334837234862,
7.52368670026048));
#7679=CARTESIAN_POINT('Ctrl Pts',(0.694889984053186,-0.562420176620936,
7.56263844726097));
#7680=CARTESIAN_POINT('Ctrl Pts',(0.823996878593897,-0.192605752293447,
7.58845159102269));
#7681=CARTESIAN_POINT('Ctrl Pts',(0.824021914564924,-0.00703811992170032,
7.60133417341575));
#7682=CARTESIAN_POINT('Ctrl Pts',(0.799999065628721,0.00692558823944229,
5.30024010712383));
#7683=CARTESIAN_POINT('Ctrl Pts',(0.799974755250737,0.187114846749742,5.31274930893178));
#7684=CARTESIAN_POINT('Ctrl Pts',(0.674578200671659,0.546127076651831,5.33781512365923));
#7685=CARTESIAN_POINT('Ctrl Pts',(0.187998995393781,0.852903359039399,5.37564381521248));
#7686=CARTESIAN_POINT('Ctrl Pts',(-0.386721866921525,0.788448388841122,
5.41368605209984));
#7687=CARTESIAN_POINT('Ctrl Pts',(-0.7983994419892,0.377627224111744,5.45194644400096));
#7688=CARTESIAN_POINT('Ctrl Pts',(-0.864375113399524,-0.203617876612744,
5.49042055747836));
#7689=CARTESIAN_POINT('Ctrl Pts',(-0.552019639313923,-0.701812288635587,
5.52910737914477));
#7690=CARTESIAN_POINT('Ctrl Pts',(0.00615426428515267,-0.897757418326962,
5.56800374230524));
#7691=CARTESIAN_POINT('Ctrl Pts',(0.463089276607972,-0.737891299975203,
5.59986549204054));
#7692=CARTESIAN_POINT('Ctrl Pts',(0.706662565433678,-0.474149107376678,
5.62457829573124));
#7693=CARTESIAN_POINT('Ctrl Pts',(0.854347338563578,-0.169471123140589,
5.6478904398873));
#7694=CARTESIAN_POINT('Ctrl Pts',(0.854381411403854,0.269671075667267,5.67712918390586));
#7695=CARTESIAN_POINT('Ctrl Pts',(0.581578462406747,0.670744438556907,5.70943359497258));
#7696=CARTESIAN_POINT('Ctrl Pts',(0.189982000930166,0.858805851522918,5.73891161848027));
#7697=CARTESIAN_POINT('Ctrl Pts',(-0.201854620920769,0.859148371452269,
5.76552549972421));
#7698=CARTESIAN_POINT('Ctrl Pts',(-0.556170302204947,0.688486751453872,
5.79222147180784));
#7699=CARTESIAN_POINT('Ctrl Pts',(-0.802120584542054,0.380288702719923,
5.81899788702529));
#7700=CARTESIAN_POINT('Ctrl Pts',(-0.890321102734134,-0.0053444036833259,
5.84585301727138));
#7701=CARTESIAN_POINT('Ctrl Pts',(-0.816781798992104,-0.327577127496462,
5.86829638740099));
#7702=CARTESIAN_POINT('Ctrl Pts',(-0.678277859648778,-0.547664335405585,
5.88628859994389));
#7703=CARTESIAN_POINT('Ctrl Pts',(-0.494316135451619,-0.731945478665225,
5.90430550175064));
#7704=CARTESIAN_POINT('Ctrl Pts',(-0.194941007989142,-0.876310026230692,
5.92687230420244));
#7705=CARTESIAN_POINT('Ctrl Pts',(0.204945568353256,-0.876409485122255,
5.95402353339188));
#7706=CARTESIAN_POINT('Ctrl Pts',(0.566325487118899,-0.702556101088839,
5.98124373289334));
#7707=CARTESIAN_POINT('Ctrl Pts',(0.816751045229916,-0.388463305588866,
6.00853075028047));
#7708=CARTESIAN_POINT('Ctrl Pts',(0.917174982875959,0.0480250206861584,
6.03892142694837));
#7709=CARTESIAN_POINT('Ctrl Pts',(0.768829350780382,0.528866010776267,6.07244001895545));
#7710=CARTESIAN_POINT('Ctrl Pts',(0.338627495917749,0.872873034891815,6.10911095186911));
#7711=CARTESIAN_POINT('Ctrl Pts',(-0.212178222814091,0.914151313349766,
6.14588130840082));
#7712=CARTESIAN_POINT('Ctrl Pts',(-0.691759933067223,0.637451614256161,
6.18274515756461));
#7713=CARTESIAN_POINT('Ctrl Pts',(-0.932934482256533,0.137697594997002,
6.21969639210087));
#7714=CARTESIAN_POINT('Ctrl Pts',(-0.84730393945114,-0.435496308403701,
6.25827178793966));
#7715=CARTESIAN_POINT('Ctrl Pts',(-0.415273257958933,-0.868240176171726,
6.29847623644814));
#7716=CARTESIAN_POINT('Ctrl Pts',(0.146189896678077,-0.930950222024402,
6.33566388079779));
#7717=CARTESIAN_POINT('Ctrl Pts',(0.578787425776111,-0.722091726547751,
6.36825221458814));
#7718=CARTESIAN_POINT('Ctrl Pts',(0.835229259505866,-0.400278931762148,
6.3962159259868));
#7719=CARTESIAN_POINT('Ctrl Pts',(0.943177486850013,0.0688606453452641,
6.42887288667825));
#7720=CARTESIAN_POINT('Ctrl Pts',(0.756462512495389,0.604750444420971,6.46623690685835));
#7721=CARTESIAN_POINT('Ctrl Pts',(0.214509054547464,0.945343920852135,6.50831791566041));
#7722=CARTESIAN_POINT('Ctrl Pts',(-0.421585054233784,0.873670673138226,
6.55043539297339));
#7723=CARTESIAN_POINT('Ctrl Pts',(-0.874725713994987,0.420703846750279,
6.59257924943873));
#7724=CARTESIAN_POINT('Ctrl Pts',(-0.946491736933492,-0.216206220818672,
6.63473932973225));
#7725=CARTESIAN_POINT('Ctrl Pts',(-0.605472064685913,-0.758979181442101,
6.67690544450194));
#7726=CARTESIAN_POINT('Ctrl Pts',(-0.000509641250504898,-0.970641038681315,
6.71906739492544));
#7727=CARTESIAN_POINT('Ctrl Pts',(0.604236817182525,-0.758999928674301,
6.76121498571335));
#7728=CARTESIAN_POINT('Ctrl Pts',(0.944676427167983,-0.216670516455945,
6.80333805746961));
#7729=CARTESIAN_POINT('Ctrl Pts',(0.873719648783539,0.418956634979468,6.8454265042638));
#7730=CARTESIAN_POINT('Ctrl Pts',(0.421037273012308,0.871132652579719,6.88747029453994));
#7731=CARTESIAN_POINT('Ctrl Pts',(-0.142342851291253,0.933831870869633,
6.92479402146672));
#7732=CARTESIAN_POINT('Ctrl Pts',(-0.575104466317865,0.724476767443434,
6.95741054274359));
#7733=CARTESIAN_POINT('Ctrl Pts',(-0.831597121038275,0.403171008458228,
6.98533606563364));
#7734=CARTESIAN_POINT('Ctrl Pts',(-0.922808904665035,0.00254068286457492,
7.01322724854536));
#7735=CARTESIAN_POINT('Ctrl Pts',(-0.831484359832733,-0.397369041930912,
7.04108128388358));
#7736=CARTESIAN_POINT('Ctrl Pts',(-0.576024516479058,-0.717622866946566,
7.06889539860548));
#7737=CARTESIAN_POINT('Ctrl Pts',(-0.207464718971416,-0.895095126308869,
7.09666685370961));
#7738=CARTESIAN_POINT('Ctrl Pts',(0.200869050822812,-0.894893573965507,
7.12439296344474));
#7739=CARTESIAN_POINT('Ctrl Pts',(0.568135301656786,-0.717941543510051,
7.15207107099507));
#7740=CARTESIAN_POINT('Ctrl Pts',(0.821742493579341,-0.399813712939291,
7.17969857736332));
#7741=CARTESIAN_POINT('Ctrl Pts',(0.912100647381109,-0.00372699171446918,
7.20727292857109));
#7742=CARTESIAN_POINT('Ctrl Pts',(0.821667160899362,0.391120281113409,7.23479162069698));
#7743=CARTESIAN_POINT('Ctrl Pts',(0.527798142032111,0.760706416566583,7.26682897888736));
#7744=CARTESIAN_POINT('Ctrl Pts',(0.00437094025093319,0.944184514671381,
7.30334225024583));
#7745=CARTESIAN_POINT('Ctrl Pts',(-0.583164611559206,0.738086874931468,
7.3442757526392));
#7746=CARTESIAN_POINT('Ctrl Pts',(-0.912546668924433,0.213026529714121,
7.38505770065783));
#7747=CARTESIAN_POINT('Ctrl Pts',(-0.843060529623956,-0.400706652853849,
7.42568118182012));
#7748=CARTESIAN_POINT('Ctrl Pts',(-0.407835437985135,-0.835237258109269,
7.46613873367218));
#7749=CARTESIAN_POINT('Ctrl Pts',(0.200737244244076,-0.903598468057941,
7.5064251969444));
#7750=CARTESIAN_POINT('Ctrl Pts',(0.71672352100227,-0.578479045751934,7.54653146106904));
#7751=CARTESIAN_POINT('Ctrl Pts',(0.849917343436364,-0.197265324952655,
7.57314919120958));
#7752=CARTESIAN_POINT('Ctrl Pts',(0.849943147209423,-0.00600671278230411,
7.58642685605973));
#7753=CARTESIAN_POINT('',(0.799999065628721,0.00692558823944227,5.30024010712383));
#7754=CARTESIAN_POINT('Origin',(0.8,-5.53479071733669E-17,5.4));
#7755=CARTESIAN_POINT('',(0.849943147209423,-0.00600671278230414,7.58642685605973));
#7756=CARTESIAN_POINT('Ctrl Pts',(0.799999065628721,0.00692558823944229,
5.30024010712383));
#7757=CARTESIAN_POINT('Ctrl Pts',(0.799974755250737,0.187114846749742,5.31274930893178));
#7758=CARTESIAN_POINT('Ctrl Pts',(0.674578200671659,0.546127076651831,5.33781512365923));
#7759=CARTESIAN_POINT('Ctrl Pts',(0.187998995393781,0.852903359039399,5.37564381521248));
#7760=CARTESIAN_POINT('Ctrl Pts',(-0.386721866921525,0.788448388841122,
5.41368605209984));
#7761=CARTESIAN_POINT('Ctrl Pts',(-0.7983994419892,0.377627224111744,5.45194644400096));
#7762=CARTESIAN_POINT('Ctrl Pts',(-0.864375113399524,-0.203617876612744,
5.49042055747836));
#7763=CARTESIAN_POINT('Ctrl Pts',(-0.552019639313923,-0.701812288635587,
5.52910737914477));
#7764=CARTESIAN_POINT('Ctrl Pts',(0.00615426428515267,-0.897757418326962,
5.56800374230524));
#7765=CARTESIAN_POINT('Ctrl Pts',(0.463089276607972,-0.737891299975203,
5.59986549204054));
#7766=CARTESIAN_POINT('Ctrl Pts',(0.706662565433678,-0.474149107376678,
5.62457829573124));
#7767=CARTESIAN_POINT('Ctrl Pts',(0.854347338563578,-0.169471123140589,
5.6478904398873));
#7768=CARTESIAN_POINT('Ctrl Pts',(0.854381411403854,0.269671075667267,5.67712918390586));
#7769=CARTESIAN_POINT('Ctrl Pts',(0.581578462406747,0.670744438556907,5.70943359497258));
#7770=CARTESIAN_POINT('Ctrl Pts',(0.189982000930166,0.858805851522918,5.73891161848027));
#7771=CARTESIAN_POINT('Ctrl Pts',(-0.201854620920769,0.859148371452269,
5.76552549972421));
#7772=CARTESIAN_POINT('Ctrl Pts',(-0.556170302204947,0.688486751453872,
5.79222147180784));
#7773=CARTESIAN_POINT('Ctrl Pts',(-0.802120584542054,0.380288702719923,
5.81899788702529));
#7774=CARTESIAN_POINT('Ctrl Pts',(-0.890321102734134,-0.0053444036833259,
5.84585301727138));
#7775=CARTESIAN_POINT('Ctrl Pts',(-0.816781798992104,-0.327577127496462,
5.86829638740099));
#7776=CARTESIAN_POINT('Ctrl Pts',(-0.678277859648778,-0.547664335405585,
5.88628859994389));
#7777=CARTESIAN_POINT('Ctrl Pts',(-0.494316135451619,-0.731945478665225,
5.90430550175064));
#7778=CARTESIAN_POINT('Ctrl Pts',(-0.194941007989142,-0.876310026230692,
5.92687230420244));
#7779=CARTESIAN_POINT('Ctrl Pts',(0.204945568353256,-0.876409485122255,
5.95402353339188));
#7780=CARTESIAN_POINT('Ctrl Pts',(0.566325487118899,-0.702556101088839,
5.98124373289334));
#7781=CARTESIAN_POINT('Ctrl Pts',(0.816751045229916,-0.388463305588866,
6.00853075028047));
#7782=CARTESIAN_POINT('Ctrl Pts',(0.917174982875959,0.0480250206861584,
6.03892142694837));
#7783=CARTESIAN_POINT('Ctrl Pts',(0.768829350780382,0.528866010776267,6.07244001895545));
#7784=CARTESIAN_POINT('Ctrl Pts',(0.338627495917749,0.872873034891815,6.10911095186911));
#7785=CARTESIAN_POINT('Ctrl Pts',(-0.212178222814091,0.914151313349766,
6.14588130840082));
#7786=CARTESIAN_POINT('Ctrl Pts',(-0.691759933067223,0.637451614256161,
6.18274515756461));
#7787=CARTESIAN_POINT('Ctrl Pts',(-0.932934482256533,0.137697594997002,
6.21969639210087));
#7788=CARTESIAN_POINT('Ctrl Pts',(-0.84730393945114,-0.435496308403701,
6.25827178793966));
#7789=CARTESIAN_POINT('Ctrl Pts',(-0.415273257958933,-0.868240176171726,
6.29847623644814));
#7790=CARTESIAN_POINT('Ctrl Pts',(0.146189896678077,-0.930950222024402,
6.33566388079779));
#7791=CARTESIAN_POINT('Ctrl Pts',(0.578787425776111,-0.722091726547751,
6.36825221458814));
#7792=CARTESIAN_POINT('Ctrl Pts',(0.835229259505866,-0.400278931762148,
6.3962159259868));
#7793=CARTESIAN_POINT('Ctrl Pts',(0.943177486850013,0.0688606453452641,
6.42887288667825));
#7794=CARTESIAN_POINT('Ctrl Pts',(0.756462512495389,0.604750444420971,6.46623690685835));
#7795=CARTESIAN_POINT('Ctrl Pts',(0.214509054547464,0.945343920852135,6.50831791566041));
#7796=CARTESIAN_POINT('Ctrl Pts',(-0.421585054233784,0.873670673138226,
6.55043539297339));
#7797=CARTESIAN_POINT('Ctrl Pts',(-0.874725713994987,0.420703846750279,
6.59257924943873));
#7798=CARTESIAN_POINT('Ctrl Pts',(-0.946491736933492,-0.216206220818672,
6.63473932973225));
#7799=CARTESIAN_POINT('Ctrl Pts',(-0.605472064685913,-0.758979181442101,
6.67690544450194));
#7800=CARTESIAN_POINT('Ctrl Pts',(-0.000509641250504898,-0.970641038681315,
6.71906739492544));
#7801=CARTESIAN_POINT('Ctrl Pts',(0.604236817182525,-0.758999928674301,
6.76121498571335));
#7802=CARTESIAN_POINT('Ctrl Pts',(0.944676427167983,-0.216670516455945,
6.80333805746961));
#7803=CARTESIAN_POINT('Ctrl Pts',(0.873719648783539,0.418956634979468,6.8454265042638));
#7804=CARTESIAN_POINT('Ctrl Pts',(0.421037273012308,0.871132652579719,6.88747029453994));
#7805=CARTESIAN_POINT('Ctrl Pts',(-0.142342851291253,0.933831870869633,
6.92479402146672));
#7806=CARTESIAN_POINT('Ctrl Pts',(-0.575104466317865,0.724476767443434,
6.95741054274359));
#7807=CARTESIAN_POINT('Ctrl Pts',(-0.831597121038275,0.403171008458228,
6.98533606563364));
#7808=CARTESIAN_POINT('Ctrl Pts',(-0.922808904665035,0.00254068286457492,
7.01322724854536));
#7809=CARTESIAN_POINT('Ctrl Pts',(-0.831484359832733,-0.397369041930912,
7.04108128388358));
#7810=CARTESIAN_POINT('Ctrl Pts',(-0.576024516479058,-0.717622866946566,
7.06889539860548));
#7811=CARTESIAN_POINT('Ctrl Pts',(-0.207464718971416,-0.895095126308869,
7.09666685370961));
#7812=CARTESIAN_POINT('Ctrl Pts',(0.200869050822812,-0.894893573965507,
7.12439296344474));
#7813=CARTESIAN_POINT('Ctrl Pts',(0.568135301656786,-0.717941543510051,
7.15207107099507));
#7814=CARTESIAN_POINT('Ctrl Pts',(0.821742493579341,-0.399813712939291,
7.17969857736332));
#7815=CARTESIAN_POINT('Ctrl Pts',(0.912100647381109,-0.00372699171446918,
7.20727292857109));
#7816=CARTESIAN_POINT('Ctrl Pts',(0.821667160899362,0.391120281113409,7.23479162069698));
#7817=CARTESIAN_POINT('Ctrl Pts',(0.527798142032111,0.760706416566583,7.26682897888736));
#7818=CARTESIAN_POINT('Ctrl Pts',(0.00437094025093319,0.944184514671381,
7.30334225024583));
#7819=CARTESIAN_POINT('Ctrl Pts',(-0.583164611559206,0.738086874931468,
7.3442757526392));
#7820=CARTESIAN_POINT('Ctrl Pts',(-0.912546668924433,0.213026529714121,
7.38505770065783));
#7821=CARTESIAN_POINT('Ctrl Pts',(-0.843060529623956,-0.400706652853849,
7.42568118182012));
#7822=CARTESIAN_POINT('Ctrl Pts',(-0.407835437985135,-0.835237258109269,
7.46613873367218));
#7823=CARTESIAN_POINT('Ctrl Pts',(0.200737244244076,-0.903598468057941,
7.5064251969444));
#7824=CARTESIAN_POINT('Ctrl Pts',(0.71672352100227,-0.578479045751934,7.54653146106904));
#7825=CARTESIAN_POINT('Ctrl Pts',(0.849917343436364,-0.197265324952655,
7.57314919120958));
#7826=CARTESIAN_POINT('Ctrl Pts',(0.849943147209423,-0.00600671278230411,
7.58642685605973));
#7827=CARTESIAN_POINT('Origin',(0.799999999999999,-1.22124532708767E-15,
7.5));
#7828=CARTESIAN_POINT('Origin',(0.799999999999999,-1.22124532708767E-15,
7.5));
#7829=CARTESIAN_POINT('Origin',(0.8,-5.53479071733669E-17,5.4));
#8390=UNCERTAINTY_MEASURE_WITH_UNIT(LENGTH_MEASURE(0.001),#8429,
'DISTANCE_ACCURACY_VALUE',
'Maximum model space distance between geometric entities at asserted c
onnectivities');
#8402=UNCERTAINTY_MEASURE_WITH_UNIT(LENGTH_MEASURE(0.001),#8429,
'DISTANCE_ACCURACY_VALUE',
'Maximum model space distance between geometric entities at asserted c
onnectivities');
#8416=(
GEOMETRIC_REPRESENTATION_CONTEXT(3)
GLOBAL_UNCERTAINTY_ASSIGNED_CONTEXT((#8390))
GLOBAL_UNIT_ASSIGNED_CONTEXT((#8429,#8431,#8432))
REPRESENTATION_CONTEXT('','3D')
);
#8428=(
GEOMETRIC_REPRESENTATION_CONTEXT(3)
GLOBAL_UNCERTAINTY_ASSIGNED_CONTEXT((#8402))
GLOBAL_UNIT_ASSIGNED_CONTEXT((#8429,#8431,#8432))
REPRESENTATION_CONTEXT('','3D')
);
#8429=(
LENGTH_UNIT()
NAMED_UNIT(*)
SI_UNIT(.CENTI.,.METRE.)
);
#8431=(
NAMED_UNIT(*)
PLANE_ANGLE_UNIT()
SI_UNIT($,.RADIAN.)
);
#8432=(
NAMED_UNIT(*)
SI_UNIT($,.STERADIAN.)
SOLID_ANGLE_UNIT()
);
#8446=SHAPE_DEFINITION_REPRESENTATION(#8471,#8527);
#8471=PRODUCT_DEFINITION_SHAPE('',$,#8553);
#8527=SHAPE_REPRESENTATION('',(#4237),#8416);
#8539=PRODUCT_DEFINITION_CONTEXT('part definition',#8616,'design');
#8553=PRODUCT_DEFINITION('Control spring','Control spring',#8578,
#8539);
#8578=PRODUCT_DEFINITION_FORMATION('',$,#8631);
#8616=APPLICATION_CONTEXT(
'Core Data for Automotive Mechanical Design Process');
#8617=PRODUCT_CONTEXT('part definition',#8616,'mechanical');
#8631=PRODUCT('Control spring','Control spring',
'Control spring',(#8617));
#8699=COLOUR_RGB('Grey',0.48,0.52,0.57);
#8700=FILL_AREA_STYLE_COLOUR('',#8699);
#8701=FILL_AREA_STYLE('',(#8700));
#8702=SURFACE_STYLE_FILL_AREA(#8701);
#8703=SURFACE_SIDE_STYLE('',(#8702));
#8704=SURFACE_STYLE_USAGE(.BOTH.,#8703);
#8705=PRESENTATION_STYLE_ASSIGNMENT((#8704));
ENDSEC;
END-ISO-10303-21;
